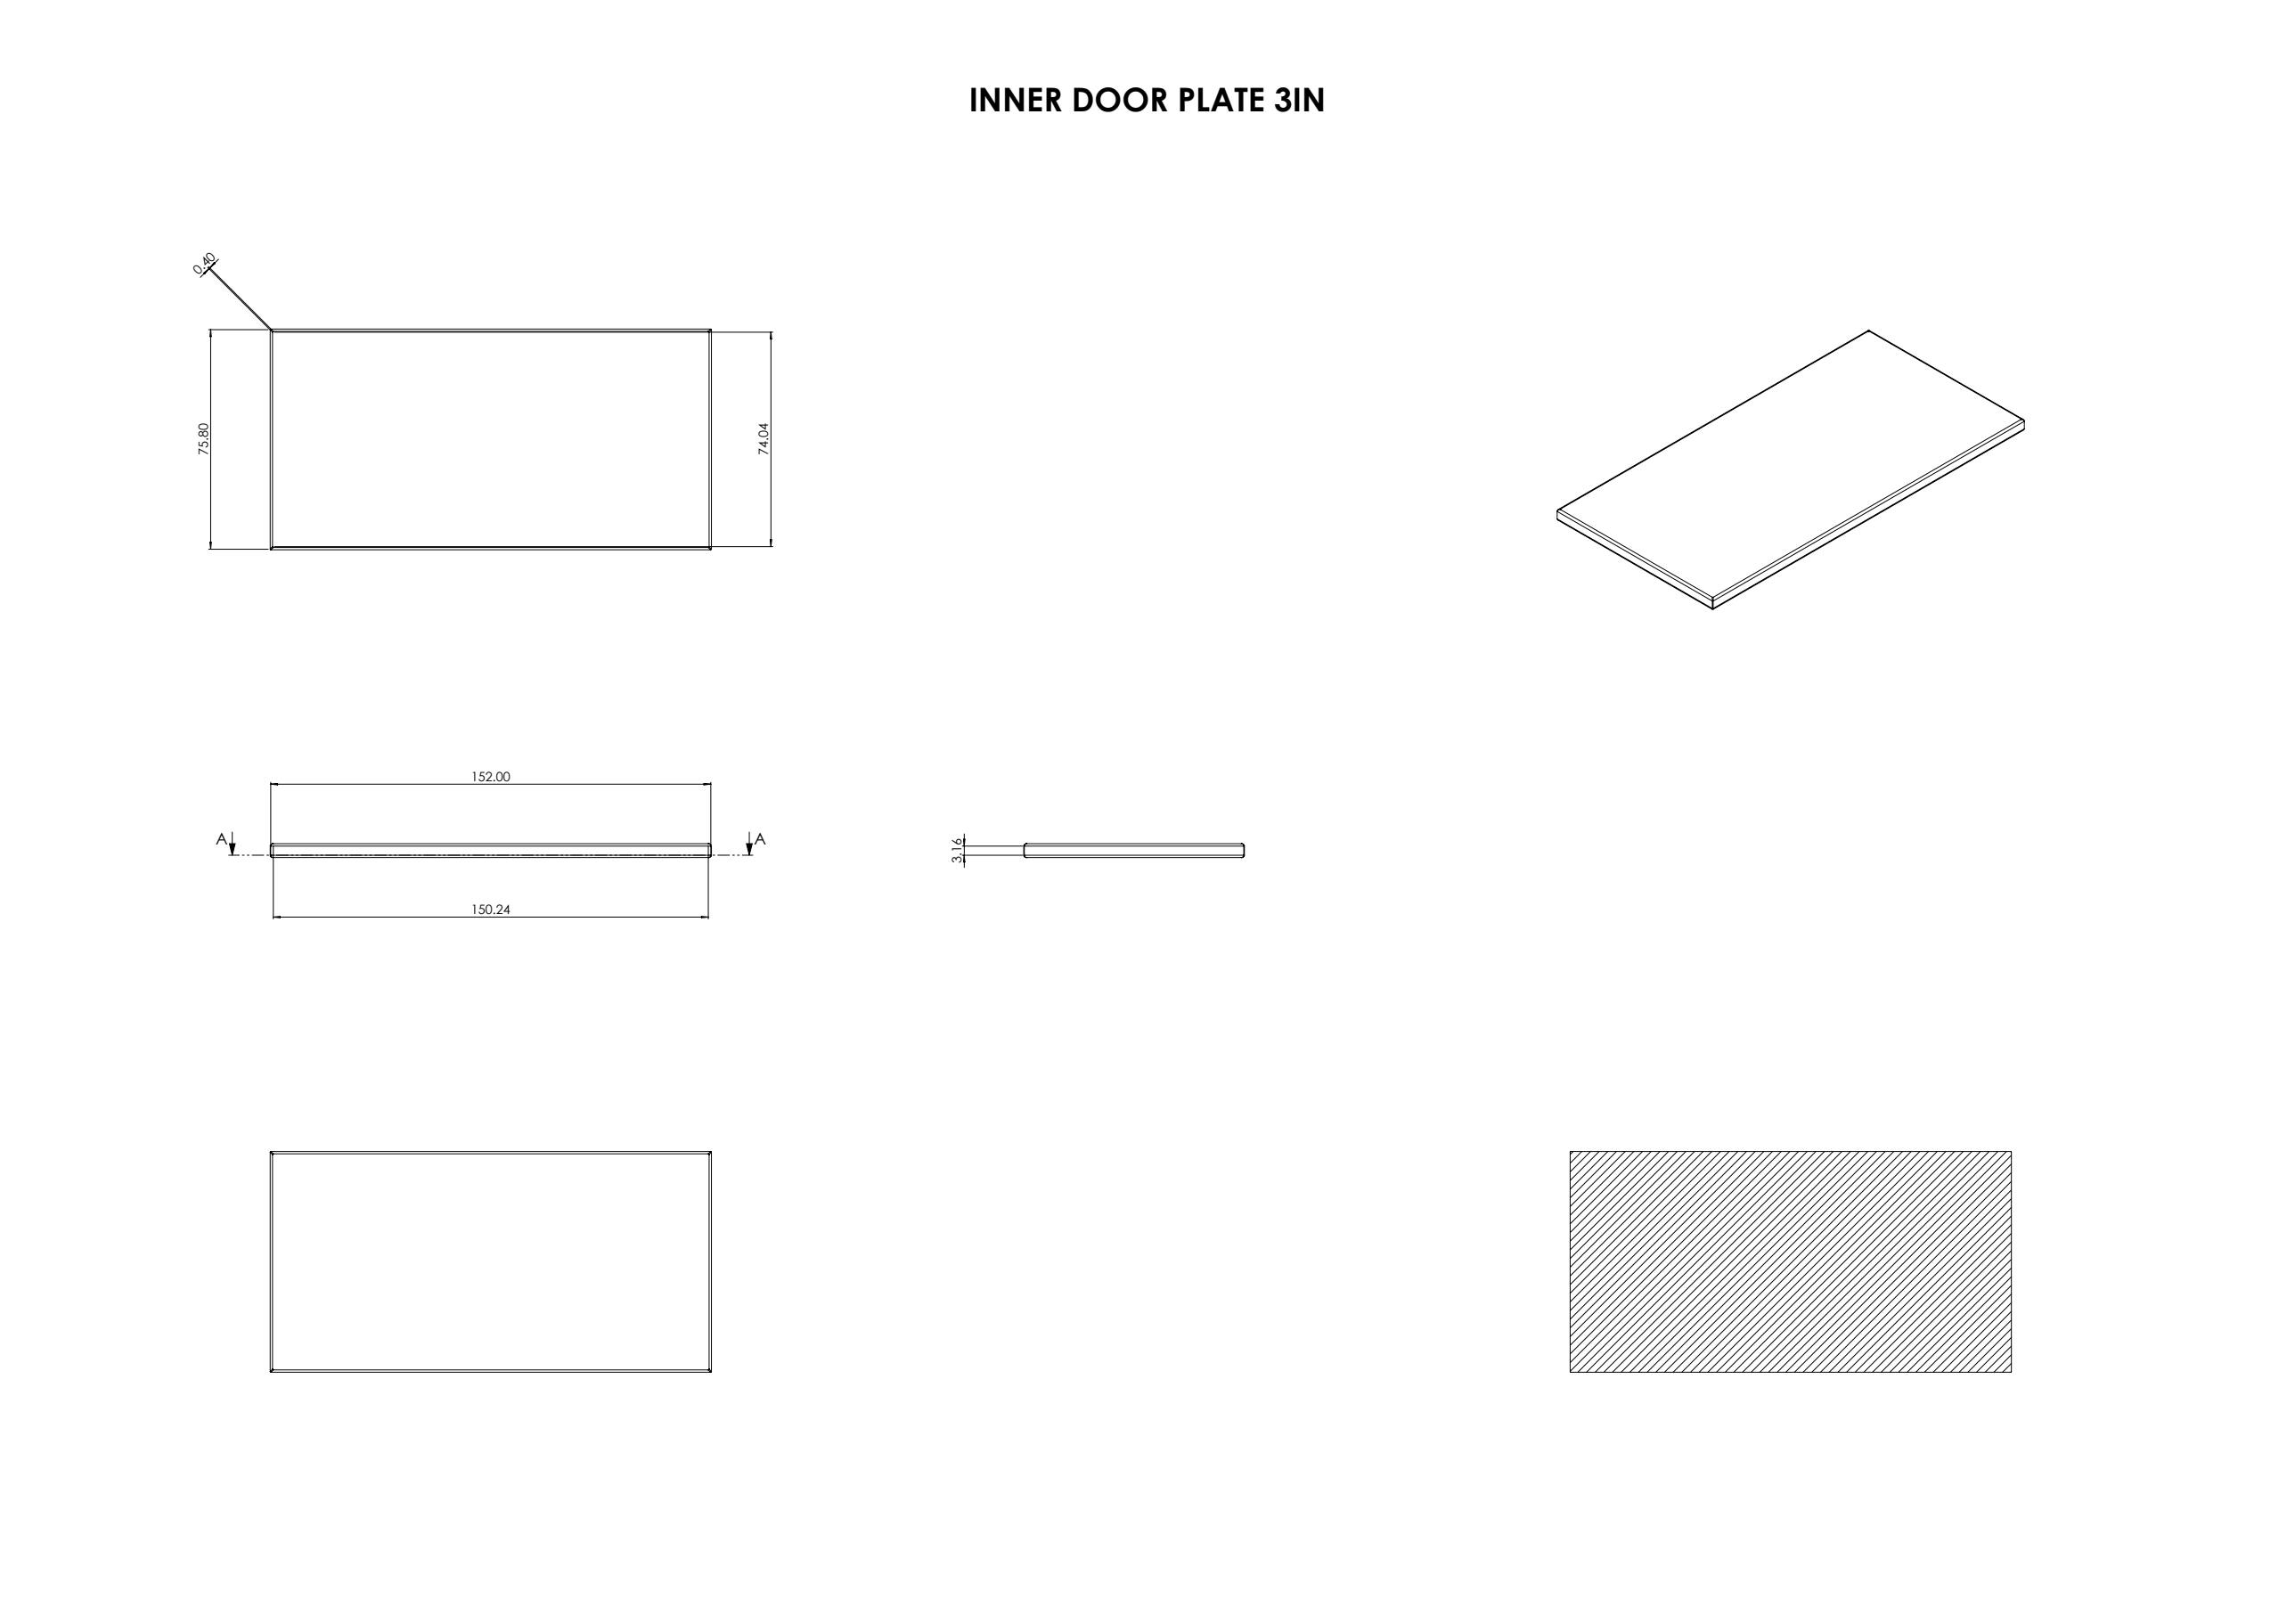
ISO-10303-21;
HEADER;
/* Generated by software containing ST-Developer
 * from STEP Tools, Inc. (www.steptools.com) 
 */

FILE_DESCRIPTION(
/* description */ (''),
/* implementation_level */ '2;1');

FILE_NAME(
/* name */ '07_Inner_Door_Plate_3in.step',
/* time_stamp */ '2026-10-25T01:30:15-07:00',
/* author */ (''),
/* organization */ (''),
/* preprocessor_version */ 'ST-DEVELOPER v20.2',
/* originating_system */ 'Autodesk Translation Framework v15.15.0.0',
/* authorisation */ '');

FILE_SCHEMA (('AUTOMOTIVE_DESIGN { 1 0 10303 214 3 1 1 }'));
ENDSEC;

DATA;
#10=MECHANICAL_DESIGN_GEOMETRIC_PRESENTATION_REPRESENTATION('',(#569),#32309);
#256=B_SPLINE_CURVE_WITH_KNOTS('',3,(#24603,#24604,#24605,#24606,#24607,
#24608,#24609,#24610,#24611,#24612,#24613,#24614,#24615,#24616,#24617,#24618,
#24619,#24620,#24621,#24622,#24623,#24624,#24625,#24626,#24627,#24628,#24629,
#24630,#24631,#24632,#24633,#24634,#24635,#24636,#24637,#24638,#24639,#24640,
#24641,#24642,#24643,#24644,#24645,#24646,#24647,#24648),.UNSPECIFIED.,
 .F.,.F.,(4,3,3,3,3,3,3,3,3,3,3,3,3,3,3,4),(0.,0.0572017311997757,0.120330894890292,
0.190833525219608,0.280000607593217,0.370000531644065,0.437396979145379,
0.498588004507602,0.56260087801746,0.634065239574647,0.727489847395828,
0.803842080523512,0.870326860317577,0.931777978339434,0.988871097236517,
1.),.UNSPECIFIED.);
#257=B_SPLINE_CURVE_WITH_KNOTS('',3,(#24650,#24651,#24652,#24653),
 .UNSPECIFIED.,.F.,.F.,(4,4),(-1.,0.),.UNSPECIFIED.);
#258=B_SPLINE_CURVE_WITH_KNOTS('',3,(#24655,#24656,#24657,#24658,#24659,
#24660,#24661,#24662,#24663,#24664,#24665,#24666,#24667,#24668,#24669,#24670,
#24671,#24672,#24673,#24674,#24675,#24676,#24677,#24678,#24679,#24680,#24681,
#24682,#24683,#24684,#24685,#24686,#24687,#24688,#24689,#24690,#24691,#24692,
#24693,#24694,#24695,#24696,#24697,#24698,#24699,#24700),.UNSPECIFIED.,
 .F.,.F.,(4,3,3,3,3,3,3,3,3,3,3,3,3,3,3,4),(0.,0.057203025224468,0.120333802338101,
0.190838689067532,0.280011837452007,0.370010357770506,0.437406670172117,
0.498598114794378,0.562610573319897,0.63407537003659,0.727505599643409,
0.803852814253569,0.870334971678201,0.931784146571509,0.988875797228613,
1.),.UNSPECIFIED.);
#259=B_SPLINE_CURVE_WITH_KNOTS('',3,(#24728,#24729,#24730,#24731,#24732,
#24733,#24734,#24735,#24736,#24737,#24738,#24739,#24740,#24741,#24742,#24743,
#24744,#24745,#24746,#24747,#24748,#24749,#24750,#24751,#24752,#24753,#24754,
#24755,#24756,#24757,#24758,#24759,#24760,#24761,#24762,#24763,#24764,#24765,
#24766,#24767,#24768,#24769,#24770,#24771,#24772,#24773),.UNSPECIFIED.,
 .F.,.F.,(4,3,3,3,3,3,3,3,3,3,3,3,3,3,3,4),(0.,0.0572017312000063,0.120330894890857,
0.190833525220496,0.280000607590238,0.370000531641458,0.437396979143437,
0.498588004432005,0.562600877937054,0.634065239482155,0.727489847253419,
0.803842080404544,0.870326860202434,0.931777978231419,0.98887109713731,
1.),.UNSPECIFIED.);
#260=B_SPLINE_CURVE_WITH_KNOTS('',3,(#24775,#24776,#24777,#24778),
 .UNSPECIFIED.,.F.,.F.,(4,4),(0.,1.),.UNSPECIFIED.);
#261=B_SPLINE_CURVE_WITH_KNOTS('',3,(#24780,#24781,#24782,#24783,#24784,
#24785,#24786,#24787,#24788,#24789,#24790,#24791,#24792,#24793,#24794,#24795,
#24796,#24797,#24798,#24799,#24800,#24801,#24802,#24803,#24804,#24805,#24806,
#24807,#24808,#24809,#24810,#24811,#24812,#24813,#24814,#24815,#24816,#24817,
#24818,#24819,#24820,#24821,#24822,#24823,#24824,#24825),.UNSPECIFIED.,
 .F.,.F.,(4,3,3,3,3,3,3,3,3,3,3,3,3,3,3,4),(0.,0.0572030252319667,0.120333802345375,
0.190838689076385,0.280011837453422,0.370010357771744,0.437406670174618,
0.498598114865344,0.562610573396659,0.634075370121406,0.727505599797859,
0.803852814376215,0.870334971791533,0.931784146677532,0.988875797332666,
1.),.UNSPECIFIED.);
#262=B_SPLINE_CURVE_WITH_KNOTS('',3,(#24852,#24853,#24854,#24855,#24856,
#24857),.UNSPECIFIED.,.F.,.F.,(4,1,1,4),(-1.70953476876622,-0.976877010723551,
-0.48843850536177,1.11854969730985E-14),.UNSPECIFIED.);
#263=B_SPLINE_CURVE_WITH_KNOTS('',3,(#24860,#24861,#24862,#24863,#24864,
#24865),.UNSPECIFIED.,.F.,.F.,(4,1,1,4),(-1.11854969730985E-14,0.48843850536177,
0.976877010723551,1.70953476876622),.UNSPECIFIED.);
#264=B_SPLINE_CURVE_WITH_KNOTS('',3,(#24900,#24901,#24902,#24903,#24904,
#24905,#24906),.UNSPECIFIED.,.F.,.F.,(4,1,1,1,4),(1.43205788482356,1.92049639018535,
2.40893489554713,2.77526377456847,3.1415926535898),.UNSPECIFIED.);
#265=B_SPLINE_CURVE_WITH_KNOTS('',3,(#24907,#24908,#24909,#24910,#24911,
#24912,#24913),.UNSPECIFIED.,.F.,.F.,(4,1,1,1,4),(-3.1415926535898,-2.77526377456847,
-2.40893489554713,-1.92049639018535,-1.43205788482356),.UNSPECIFIED.);
#266=B_SPLINE_CURVE_WITH_KNOTS('',3,(#24932,#24933,#24934,#24935,#24936,
#24937),.UNSPECIFIED.,.F.,.F.,(4,1,1,4),(-1.70953476876624,-0.976877010723567,
-0.488438505361783,0.),.UNSPECIFIED.);
#267=B_SPLINE_CURVE_WITH_KNOTS('',3,(#24938,#24939,#24940,#24941,#24942,
#24943,#24944,#24945,#24946,#24947,#24948,#24949,#24950,#24951,#24952,#24953,
#24954,#24955,#24956,#24957,#24958,#24959,#24960,#24961,#24962,#24963,#24964,
#24965,#24966,#24967,#24968,#24969,#24970,#24971,#24972,#24973,#24974,#24975,
#24976,#24977,#24978,#24979,#24980,#24981,#24982,#24983),.UNSPECIFIED.,
 .F.,.F.,(4,3,3,3,3,3,3,3,3,3,3,3,3,3,3,4),(0.,0.0572017311994344,0.120330894888931,
0.19083352521961,0.28000060759744,0.37000053164776,0.437396979149183,0.498588004127736,
0.562600877612139,0.634065239106159,0.727489846545216,0.803842079829981,
0.870326859689392,0.93177797774672,0.988871096661088,1.),.UNSPECIFIED.);
#268=B_SPLINE_CURVE_WITH_KNOTS('',3,(#24992,#24993,#24994,#24995,#24996,
#24997,#24998,#24999,#25000,#25001,#25002,#25003,#25004,#25005,#25006,#25007,
#25008,#25009,#25010,#25011,#25012,#25013,#25014,#25015,#25016,#25017,#25018,
#25019,#25020,#25021,#25022,#25023,#25024,#25025,#25026,#25027,#25028,#25029,
#25030,#25031,#25032,#25033,#25034,#25035,#25036,#25037),.UNSPECIFIED.,
 .F.,.F.,(4,3,3,3,3,3,3,3,3,3,3,3,3,3,3,4),(0.,0.0572030252313222,0.120333802345085,
0.190838689078026,0.280011837457414,0.370010357775237,0.437406670179801,
0.498598114642262,0.562610573159454,0.634075369847749,0.727505599310812,
0.803852813978605,0.870334971432735,0.931784146343715,0.988875797008993,
1.),.UNSPECIFIED.);
#269=B_SPLINE_CURVE_WITH_KNOTS('',3,(#25038,#25039,#25040,#25041,#25042,
#25043),.UNSPECIFIED.,.F.,.F.,(4,1,1,4),(0.,0.488438505361777,0.976877010723555,
1.70953476876622),.UNSPECIFIED.);
#270=B_SPLINE_CURVE_WITH_KNOTS('',3,(#25070,#25071,#25072,#25073,#25074,
#25075,#25076,#25077,#25078,#25079,#25080,#25081,#25082,#25083,#25084,#25085,
#25086,#25087,#25088,#25089,#25090,#25091,#25092,#25093,#25094,#25095,#25096,
#25097,#25098,#25099,#25100,#25101,#25102,#25103,#25104,#25105,#25106,#25107,
#25108,#25109,#25110,#25111,#25112,#25113,#25114,#25115),.UNSPECIFIED.,
 .F.,.F.,(4,3,3,3,3,3,3,3,3,3,3,3,3,3,3,4),(0.,0.0572017311976094,0.120330894887026,
0.190833525221234,0.280000607599086,0.3700005316492,0.437396979153787,0.498588004443689,
0.562600877950485,0.634065239495553,0.727489847237366,0.803842080393393,
0.87032686020045,0.931777978227553,0.988871097128439,1.),.UNSPECIFIED.);
#271=B_SPLINE_CURVE_WITH_KNOTS('',3,(#25116,#25117,#25118,#25119),
 .UNSPECIFIED.,.F.,.F.,(4,4),(0.,1.),.UNSPECIFIED.);
#272=B_SPLINE_CURVE_WITH_KNOTS('',3,(#25146,#25147,#25148,#25149),
 .UNSPECIFIED.,.F.,.F.,(4,4),(0.,1.),.UNSPECIFIED.);
#273=B_SPLINE_CURVE_WITH_KNOTS('',3,(#25150,#25151,#25152,#25153,#25154,
#25155,#25156,#25157,#25158,#25159,#25160,#25161,#25162,#25163,#25164,#25165,
#25166,#25167,#25168,#25169,#25170,#25171,#25172,#25173,#25174,#25175,#25176,
#25177,#25178,#25179,#25180,#25181,#25182,#25183,#25184,#25185,#25186,#25187,
#25188,#25189,#25190,#25191,#25192,#25193,#25194,#25195),.UNSPECIFIED.,
 .F.,.F.,(4,3,3,3,3,3,3,3,3,3,3,3,3,3,3,4),(0.,0.0572030252324622,0.120333802346723,
0.190838689076922,0.280011837457471,0.370010357775287,0.437406670183435,
0.498598114641987,0.562610573159151,0.634075369845933,0.727505599300381,
0.803852813971137,0.870334971421258,0.931784146332158,0.988875796999179,
1.),.UNSPECIFIED.);
#274=B_SPLINE_CURVE_WITH_KNOTS('',3,(#25222,#25223,#25224,#25225,#25226,
#25227),.UNSPECIFIED.,.F.,.F.,(4,1,1,4),(0.,0.488438505361783,0.976877010723567,
1.70953476876624),.UNSPECIFIED.);
#275=B_SPLINE_CURVE_WITH_KNOTS('',3,(#25256,#25257,#25258,#25259,#25260,
#25261),.UNSPECIFIED.,.F.,.F.,(4,1,1,4),(-1.70953476876622,-0.976877010723555,
-0.488438505361777,0.),.UNSPECIFIED.);
#276=B_SPLINE_CURVE_WITH_KNOTS('',3,(#25287,#25288,#25289,#25290,#25291,
#25292,#25293,#25294,#25295,#25296,#25297,#25298,#25299,#25300,#25301,#25302,
#25303,#25304,#25305,#25306,#25307,#25308,#25309,#25310,#25311,#25312,#25313,
#25314,#25315,#25316,#25317,#25318,#25319,#25320,#25321,#25322,#25323,#25324,
#25325,#25326,#25327,#25328,#25329,#25330,#25331,#25332),.UNSPECIFIED.,
 .F.,.F.,(4,3,3,3,3,3,3,3,3,3,3,3,3,3,3,4),(0.,0.0572017311991183,0.120330894889653,
0.190833525219955,0.280000607594411,0.37000053164511,0.437396979144203,
0.498588004649256,0.56260087816826,0.634065239749291,0.727489847706123,
0.803842080776209,0.870326860547973,0.931777978552727,0.988871097444316,
1.),.UNSPECIFIED.);
#277=B_SPLINE_CURVE_WITH_KNOTS('',3,(#25334,#25335,#25336,#25337),
 .UNSPECIFIED.,.F.,.F.,(4,4),(0.,1.),.UNSPECIFIED.);
#278=B_SPLINE_CURVE_WITH_KNOTS('',3,(#25338,#25339,#25340,#25341,#25342,
#25343,#25344,#25345,#25346,#25347,#25348,#25349,#25350,#25351,#25352,#25353,
#25354,#25355,#25356,#25357,#25358,#25359,#25360,#25361,#25362,#25363,#25364,
#25365,#25366,#25367,#25368,#25369,#25370,#25371,#25372,#25373,#25374,#25375,
#25376,#25377,#25378,#25379,#25380,#25381,#25382,#25383),.UNSPECIFIED.,
 .F.,.F.,(4,3,3,3,3,3,3,3,3,3,3,3,3,3,3,4),(0.,0.0572030252343024,0.12033380234866,
0.190838689076873,0.280011837448138,0.370010357767121,0.437406670172275,
0.498598114697011,0.562610573216881,0.634075369917583,0.727505599449089,
0.803852814091775,0.870334971532607,0.931784146442687,0.988875797099411,
1.),.UNSPECIFIED.);
#279=B_SPLINE_CURVE_WITH_KNOTS('',3,(#25410,#25411,#25412,#25413,#25414,
#25415,#25416,#25417,#25418,#25419,#25420,#25421,#25422,#25423,#25424,#25425,
#25426,#25427,#25428,#25429,#25430,#25431,#25432,#25433,#25434,#25435,#25436,
#25437,#25438,#25439,#25440,#25441,#25442,#25443,#25444,#25445,#25446,#25447,
#25448,#25449,#25450,#25451,#25452,#25453,#25454,#25455),.UNSPECIFIED.,
 .F.,.F.,(4,3,3,3,3,3,3,3,3,3,3,3,3,3,3,4),(0.,0.0572017312009936,0.120330894888744,
0.190833525225305,0.280000607597786,0.370000531648063,0.437396979151322,
0.49858800483577,0.562600878367579,0.634065239978569,0.727489848107998,
0.8038420811056,0.870326860843456,0.931777978817204,0.988871097702708,1.),
 .UNSPECIFIED.);
#280=B_SPLINE_CURVE_WITH_KNOTS('',3,(#25457,#25458,#25459,#25460),
 .UNSPECIFIED.,.F.,.F.,(4,4),(0.,1.),.UNSPECIFIED.);
#281=B_SPLINE_CURVE_WITH_KNOTS('',3,(#25462,#25463,#25464,#25465,#25466,
#25467,#25468,#25469,#25470,#25471,#25472,#25473,#25474,#25475,#25476,#25477,
#25478,#25479,#25480,#25481,#25482,#25483,#25484,#25485,#25486,#25487,#25488,
#25489,#25490,#25491,#25492,#25493,#25494,#25495,#25496,#25497,#25498,#25499,
#25500,#25501,#25502,#25503,#25504,#25505,#25506,#25507),.UNSPECIFIED.,
 .F.,.F.,(4,3,3,3,3,3,3,3,3,3,3,3,3,3,3,4),(0.,0.0572030252317164,0.120333802345145,
0.19083868907559,0.280011837455817,0.37001035777384,0.437406670175968,0.498598114641638,
0.562610573158253,0.634075369846188,0.727505599314327,0.803852813981206,
0.870334971433397,0.93178414634131,0.98887579700713,1.),.UNSPECIFIED.);
#282=B_SPLINE_CURVE_WITH_KNOTS('',3,(#25534,#25535,#25536,#25537,#25538,
#25539),.UNSPECIFIED.,.F.,.F.,(4,1,1,4),(-1.70953476876621,-0.976877010723542,
-0.48843850536176,2.22044604925035E-14),.UNSPECIFIED.);
#283=B_SPLINE_CURVE_WITH_KNOTS('',3,(#25542,#25543,#25544,#25545,#25546,
#25547),.UNSPECIFIED.,.F.,.F.,(4,1,1,4),(-2.22044604925035E-14,0.48843850536176,
0.976877010723542,1.70953476876621),.UNSPECIFIED.);
#284=B_SPLINE_CURVE_WITH_KNOTS('',3,(#25578,#25579,#25580,#25581,#25582,
#25583),.UNSPECIFIED.,.F.,.F.,(4,1,1,4),(-1.70953476876621,-0.97687701072354,
-0.488438505361759,2.22044604925031E-14),.UNSPECIFIED.);
#285=B_SPLINE_CURVE_WITH_KNOTS('',3,(#25584,#25585,#25586,#25587,#25588,
#25589),.UNSPECIFIED.,.F.,.F.,(4,1,1,4),(-2.22044604925031E-14,0.488438505361759,
0.97687701072354,1.70953476876621),.UNSPECIFIED.);
#286=B_SPLINE_CURVE_WITH_KNOTS('',3,(#25594,#25595,#25596,#25597,#25598,
#25599),.UNSPECIFIED.,.F.,.F.,(4,1,1,4),(-1.70953476876623,-0.976877010723559,
-0.488438505361781,-2.77555756156289E-15),.UNSPECIFIED.);
#287=B_SPLINE_CURVE_WITH_KNOTS('',3,(#25600,#25601,#25602,#25603,#25604,
#25605,#25606,#25607,#25608,#25609,#25610,#25611,#25612,#25613,#25614,#25615,
#25616,#25617,#25618,#25619,#25620,#25621,#25622,#25623,#25624,#25625,#25626,
#25627,#25628,#25629,#25630,#25631,#25632,#25633,#25634,#25635,#25636,#25637,
#25638,#25639,#25640,#25641,#25642,#25643,#25644,#25645),.UNSPECIFIED.,
 .F.,.F.,(4,3,3,3,3,3,3,3,3,3,3,3,3,3,3,4),(0.,0.0572017311987612,0.120330894889715,
0.190833525218877,0.280000607593098,0.370000531643961,0.437396979144952,
0.498588004371557,0.562600877871927,0.634065239405833,0.727489847083102,
0.803842080268102,0.870326860085879,0.931777978122396,0.988871097026644,
1.),.UNSPECIFIED.);
#288=B_SPLINE_CURVE_WITH_KNOTS('',3,(#25654,#25655,#25656,#25657,#25658,
#25659,#25660,#25661,#25662,#25663,#25664,#25665,#25666,#25667,#25668,#25669,
#25670,#25671,#25672,#25673,#25674,#25675,#25676,#25677,#25678,#25679,#25680,
#25681,#25682,#25683,#25684,#25685,#25686,#25687,#25688,#25689,#25690,#25691,
#25692,#25693,#25694,#25695,#25696,#25697,#25698,#25699),.UNSPECIFIED.,
 .F.,.F.,(4,3,3,3,3,3,3,3,3,3,3,3,3,3,3,4),(0.,0.0572030252318266,0.120333802345496,
0.190838689075676,0.280011837456741,0.370010357774648,0.437406670177162,
0.498598114850172,0.562610573381775,0.634075370104953,0.727505599770209,
0.803852814352912,0.870334971770891,0.9317841466576,0.988875797314384,1.),
 .UNSPECIFIED.);
#289=B_SPLINE_CURVE_WITH_KNOTS('',3,(#25700,#25701,#25702,#25703,#25704,
#25705),.UNSPECIFIED.,.F.,.F.,(4,1,1,4),(2.77555756156289E-15,0.488438505361782,
0.976877010723562,1.70953476876623),.UNSPECIFIED.);
#290=B_SPLINE_CURVE_WITH_KNOTS('',3,(#25736,#25737,#25738,#25739),
 .UNSPECIFIED.,.F.,.F.,(4,4),(0.,1.),.UNSPECIFIED.);
#291=B_SPLINE_CURVE_WITH_KNOTS('',3,(#25740,#25741,#25742,#25743,#25744,
#25745,#25746,#25747,#25748,#25749,#25750,#25751,#25752,#25753,#25754,#25755,
#25756,#25757,#25758,#25759,#25760,#25761,#25762,#25763,#25764,#25765,#25766,
#25767,#25768,#25769,#25770,#25771,#25772,#25773,#25774,#25775,#25776,#25777,
#25778,#25779,#25780,#25781,#25782,#25783,#25784,#25785),.UNSPECIFIED.,
 .F.,.F.,(4,3,3,3,3,3,3,3,3,3,3,3,3,3,3,4),(0.,0.0572030252318119,0.120333802345044,
0.190838689074226,0.280011837457671,0.370010357775463,0.437406670175368,
0.498598114719374,0.562610573241369,0.634075369941395,0.727505599476499,
0.803852814114293,0.870334971552934,0.931784146453147,0.98887579711519,
1.),.UNSPECIFIED.);
#292=B_SPLINE_CURVE_WITH_KNOTS('',3,(#25811,#25812,#25813,#25814,#25815,
#25816,#25817,#25818,#25819,#25820,#25821,#25822,#25823,#25824,#25825,#25826,
#25827,#25828,#25829,#25830,#25831,#25832,#25833,#25834,#25835,#25836,#25837,
#25838,#25839,#25840,#25841,#25842,#25843,#25844,#25845,#25846,#25847,#25848,
#25849,#25850,#25851,#25852,#25853,#25854,#25855,#25856),.UNSPECIFIED.,
 .F.,.F.,(4,3,3,3,3,3,3,3,3,3,3,3,3,3,3,4),(0.,0.0572017311987599,0.120330894889451,
0.190833525224185,0.28000060760209,0.370000531651829,0.437396979150436,
0.498588004343821,0.562600877842339,0.63406523937154,0.727489847024129,
0.803842080219329,0.870326860044885,0.931777978082536,0.988871096986048,
1.),.UNSPECIFIED.);
#293=B_SPLINE_CURVE_WITH_KNOTS('',3,(#25857,#25858,#25859,#25860),
 .UNSPECIFIED.,.F.,.F.,(4,4),(0.,1.),.UNSPECIFIED.);
#294=B_SPLINE_CURVE_WITH_KNOTS('',3,(#25886,#25887,#25888,#25889,#25890,
#25891),.UNSPECIFIED.,.F.,.F.,(4,1,1,4),(-1.70953476876623,-0.976877010723562,
-0.488438505361782,-2.77555756156289E-15),.UNSPECIFIED.);
#295=B_SPLINE_CURVE_WITH_KNOTS('',3,(#25921,#25922,#25923,#25924,#25925,
#25926),.UNSPECIFIED.,.F.,.F.,(4,1,1,4),(2.77555756156289E-15,0.488438505361781,
0.976877010723559,1.70953476876623),.UNSPECIFIED.);
#471=B_SPLINE_SURFACE_WITH_KNOTS('',3,3,((#24577,#24578,#24579,#24580,#24581,
#24582),(#24583,#24584,#24585,#24586,#24587,#24588),(#24589,#24590,#24591,
#24592,#24593,#24594),(#24595,#24596,#24597,#24598,#24599,#24600)),
 .UNSPECIFIED.,.F.,.F.,.F.,(4,4),(4,1,1,4),(0.,1.),(0.,0.571428571428571,
0.857142857142857,1.),.UNSPECIFIED.);
#472=B_SPLINE_SURFACE_WITH_KNOTS('',3,3,((#24702,#24703,#24704,#24705,#24706,
#24707),(#24708,#24709,#24710,#24711,#24712,#24713),(#24714,#24715,#24716,
#24717,#24718,#24719),(#24720,#24721,#24722,#24723,#24724,#24725)),
 .UNSPECIFIED.,.F.,.F.,.F.,(4,4),(4,1,1,4),(0.,1.),(0.,0.571428571428571,
0.857142857142857,1.),.UNSPECIFIED.);
#473=B_SPLINE_SURFACE_WITH_KNOTS('',3,3,((#24827,#24828,#24829,#24830,#24831,
#24832),(#24833,#24834,#24835,#24836,#24837,#24838),(#24839,#24840,#24841,
#24842,#24843,#24844),(#24845,#24846,#24847,#24848,#24849,#24850)),
 .UNSPECIFIED.,.F.,.F.,.F.,(4,4),(4,1,1,4),(0.,1.),(-1.70953476876622,-0.976877010723551,
-0.48843850536177,1.11854969730985E-14),.UNSPECIFIED.);
#474=B_SPLINE_SURFACE_WITH_KNOTS('',3,3,((#24872,#24873,#24874,#24875,#24876,
#24877,#24878),(#24879,#24880,#24881,#24882,#24883,#24884,#24885),(#24886,
#24887,#24888,#24889,#24890,#24891,#24892),(#24893,#24894,#24895,#24896,
#24897,#24898,#24899)),.UNSPECIFIED.,.F.,.F.,.F.,(4,4),(4,1,1,1,4),(0.,
1.),(-3.1415926535898,-2.77526377456847,-2.40893489554713,-1.92049639018535,
-1.43205788482356),.UNSPECIFIED.);
#475=B_SPLINE_SURFACE_WITH_KNOTS('',3,3,((#25044,#25045,#25046,#25047,#25048,
#25049),(#25050,#25051,#25052,#25053,#25054,#25055),(#25056,#25057,#25058,
#25059,#25060,#25061),(#25062,#25063,#25064,#25065,#25066,#25067)),
 .UNSPECIFIED.,.F.,.F.,.F.,(4,4),(4,1,1,4),(0.,1.),(0.,0.571428571428571,
0.857142857142857,1.),.UNSPECIFIED.);
#476=B_SPLINE_SURFACE_WITH_KNOTS('',3,3,((#25121,#25122,#25123,#25124,#25125,
#25126),(#25127,#25128,#25129,#25130,#25131,#25132),(#25133,#25134,#25135,
#25136,#25137,#25138),(#25139,#25140,#25141,#25142,#25143,#25144)),
 .UNSPECIFIED.,.F.,.F.,.F.,(4,4),(4,1,1,4),(0.,1.),(0.,0.571428571428571,
0.857142857142857,1.),.UNSPECIFIED.);
#477=B_SPLINE_SURFACE_WITH_KNOTS('',3,3,((#25196,#25197,#25198,#25199,#25200,
#25201),(#25202,#25203,#25204,#25205,#25206,#25207),(#25208,#25209,#25210,
#25211,#25212,#25213),(#25214,#25215,#25216,#25217,#25218,#25219)),
 .UNSPECIFIED.,.F.,.F.,.F.,(4,4),(4,1,1,4),(0.,1.),(-1.70953476876624,-0.976877010723567,
-0.488438505361783,0.),.UNSPECIFIED.);
#478=B_SPLINE_SURFACE_WITH_KNOTS('',3,3,((#25232,#25233,#25234,#25235,#25236,
#25237),(#25238,#25239,#25240,#25241,#25242,#25243),(#25244,#25245,#25246,
#25247,#25248,#25249),(#25250,#25251,#25252,#25253,#25254,#25255)),
 .UNSPECIFIED.,.F.,.F.,.F.,(4,4),(4,1,1,4),(0.,1.),(-1.70953476876622,-0.976877010723555,
-0.488438505361777,0.),.UNSPECIFIED.);
#479=B_SPLINE_SURFACE_WITH_KNOTS('',3,3,((#25262,#25263,#25264,#25265,#25266,
#25267),(#25268,#25269,#25270,#25271,#25272,#25273),(#25274,#25275,#25276,
#25277,#25278,#25279),(#25280,#25281,#25282,#25283,#25284,#25285)),
 .UNSPECIFIED.,.F.,.F.,.F.,(4,4),(4,1,1,4),(0.,1.),(0.,0.571428571428571,
0.857142857142857,1.),.UNSPECIFIED.);
#480=B_SPLINE_SURFACE_WITH_KNOTS('',3,3,((#25384,#25385,#25386,#25387,#25388,
#25389),(#25390,#25391,#25392,#25393,#25394,#25395),(#25396,#25397,#25398,
#25399,#25400,#25401),(#25402,#25403,#25404,#25405,#25406,#25407)),
 .UNSPECIFIED.,.F.,.F.,.F.,(4,4),(4,1,1,4),(0.,1.),(0.,0.571428571428571,
0.857142857142857,1.),.UNSPECIFIED.);
#481=B_SPLINE_SURFACE_WITH_KNOTS('',3,3,((#25509,#25510,#25511,#25512,#25513,
#25514),(#25515,#25516,#25517,#25518,#25519,#25520),(#25521,#25522,#25523,
#25524,#25525,#25526),(#25527,#25528,#25529,#25530,#25531,#25532)),
 .UNSPECIFIED.,.F.,.F.,.F.,(4,4),(4,1,1,4),(0.,1.),(-1.70953476876621,-0.976877010723542,
-0.48843850536176,2.22044604925035E-14),.UNSPECIFIED.);
#482=B_SPLINE_SURFACE_WITH_KNOTS('',3,3,((#25554,#25555,#25556,#25557,#25558,
#25559),(#25560,#25561,#25562,#25563,#25564,#25565),(#25566,#25567,#25568,
#25569,#25570,#25571),(#25572,#25573,#25574,#25575,#25576,#25577)),
 .UNSPECIFIED.,.F.,.F.,.F.,(4,4),(4,1,1,4),(0.,1.),(-1.70953476876621,-0.97687701072354,
-0.488438505361759,2.22044604925031E-14),.UNSPECIFIED.);
#483=B_SPLINE_SURFACE_WITH_KNOTS('',3,3,((#25711,#25712,#25713,#25714,#25715,
#25716),(#25717,#25718,#25719,#25720,#25721,#25722),(#25723,#25724,#25725,
#25726,#25727,#25728),(#25729,#25730,#25731,#25732,#25733,#25734)),
 .UNSPECIFIED.,.F.,.F.,.F.,(4,4),(4,1,1,4),(0.,1.),(0.,0.571428571428571,
0.857142857142857,1.),.UNSPECIFIED.);
#484=B_SPLINE_SURFACE_WITH_KNOTS('',3,3,((#25786,#25787,#25788,#25789,#25790,
#25791),(#25792,#25793,#25794,#25795,#25796,#25797),(#25798,#25799,#25800,
#25801,#25802,#25803),(#25804,#25805,#25806,#25807,#25808,#25809)),
 .UNSPECIFIED.,.F.,.F.,.F.,(4,4),(4,1,1,4),(0.,1.),(0.,0.571428571428571,
0.857142857142857,1.),.UNSPECIFIED.);
#485=B_SPLINE_SURFACE_WITH_KNOTS('',3,3,((#25861,#25862,#25863,#25864,#25865,
#25866),(#25867,#25868,#25869,#25870,#25871,#25872),(#25873,#25874,#25875,
#25876,#25877,#25878),(#25879,#25880,#25881,#25882,#25883,#25884)),
 .UNSPECIFIED.,.F.,.F.,.F.,(4,4),(4,1,1,4),(0.,1.),(-1.70953476876623,-0.976877010723562,
-0.488438505361782,-2.77555756156289E-15),.UNSPECIFIED.);
#486=B_SPLINE_SURFACE_WITH_KNOTS('',3,3,((#25897,#25898,#25899,#25900,#25901,
#25902),(#25903,#25904,#25905,#25906,#25907,#25908),(#25909,#25910,#25911,
#25912,#25913,#25914),(#25915,#25916,#25917,#25918,#25919,#25920)),
 .UNSPECIFIED.,.F.,.F.,.F.,(4,4),(4,1,1,4),(0.,1.),(-1.70953476876623,-0.976877010723559,
-0.488438505361781,-2.77555756156289E-15),.UNSPECIFIED.);
#541=SHAPE_REPRESENTATION_RELATIONSHIP('SRR','None',#32368,#555);
#555=ADVANCED_BREP_SHAPE_REPRESENTATION('',(#583),#32301);
#569=STYLED_ITEM('',(#32495),#583);
#583=MANIFOLD_SOLID_BREP('Body1',#13810);
#718=CYLINDRICAL_SURFACE('',#14416,0.8);
#719=CYLINDRICAL_SURFACE('',#14418,0.8);
#720=CYLINDRICAL_SURFACE('',#14421,0.8);
#721=CYLINDRICAL_SURFACE('',#14423,0.8);
#722=CYLINDRICAL_SURFACE('',#14426,0.8);
#723=CYLINDRICAL_SURFACE('',#14428,0.8);
#724=CYLINDRICAL_SURFACE('',#14429,0.8);
#725=CYLINDRICAL_SURFACE('',#14431,0.8);
#1561=FACE_OUTER_BOUND('',#2396,.T.);
#1562=FACE_OUTER_BOUND('',#2397,.T.);
#1563=FACE_OUTER_BOUND('',#2398,.T.);
#1564=FACE_OUTER_BOUND('',#2399,.T.);
#1565=FACE_OUTER_BOUND('',#2400,.T.);
#1566=FACE_OUTER_BOUND('',#2401,.T.);
#1567=FACE_OUTER_BOUND('',#2402,.T.);
#1568=FACE_OUTER_BOUND('',#2403,.T.);
#1569=FACE_OUTER_BOUND('',#2404,.T.);
#1570=FACE_OUTER_BOUND('',#2405,.T.);
#1571=FACE_OUTER_BOUND('',#2406,.T.);
#1572=FACE_OUTER_BOUND('',#2407,.T.);
#1573=FACE_OUTER_BOUND('',#2408,.T.);
#1574=FACE_OUTER_BOUND('',#2409,.T.);
#1575=FACE_OUTER_BOUND('',#2410,.T.);
#1576=FACE_OUTER_BOUND('',#2411,.T.);
#1577=FACE_OUTER_BOUND('',#2412,.T.);
#1578=FACE_OUTER_BOUND('',#2413,.T.);
#1579=FACE_OUTER_BOUND('',#2414,.T.);
#1580=FACE_OUTER_BOUND('',#2415,.T.);
#1581=FACE_OUTER_BOUND('',#2416,.T.);
#1582=FACE_OUTER_BOUND('',#2417,.T.);
#1583=FACE_OUTER_BOUND('',#2418,.T.);
#1584=FACE_OUTER_BOUND('',#2419,.T.);
#1585=FACE_OUTER_BOUND('',#2420,.T.);
#1586=FACE_OUTER_BOUND('',#2421,.T.);
#1587=FACE_OUTER_BOUND('',#2422,.T.);
#1588=FACE_OUTER_BOUND('',#2423,.T.);
#1589=FACE_OUTER_BOUND('',#2424,.T.);
#1590=FACE_OUTER_BOUND('',#2425,.T.);
#1591=FACE_OUTER_BOUND('',#2426,.T.);
#1592=FACE_OUTER_BOUND('',#2427,.T.);
#1593=FACE_OUTER_BOUND('',#2428,.T.);
#1594=FACE_OUTER_BOUND('',#2429,.T.);
#2396=EDGE_LOOP('',(#10209,#10210,#10211,#10212));
#2397=EDGE_LOOP('',(#10213,#10214,#10215,#10216));
#2398=EDGE_LOOP('',(#10217,#10218,#10219,#10220));
#2399=EDGE_LOOP('',(#10221,#10222,#10223,#10224));
#2400=EDGE_LOOP('',(#10225,#10226,#10227,#10228));
#2401=EDGE_LOOP('',(#10229,#10230,#10231,#10232,#10233,#10234,#10235,#10236));
#2402=EDGE_LOOP('',(#10237,#10238,#10239,#10240,#10241,#10242));
#2403=EDGE_LOOP('',(#10243,#10244,#10245,#10246));
#2404=EDGE_LOOP('',(#10247,#10248,#10249,#10250,#10251,#10252));
#2405=EDGE_LOOP('',(#10253,#10254,#10255,#10256));
#2406=EDGE_LOOP('',(#10257,#10258,#10259,#10260));
#2407=EDGE_LOOP('',(#10261,#10262,#10263,#10264));
#2408=EDGE_LOOP('',(#10265,#10266,#10267,#10268));
#2409=EDGE_LOOP('',(#10269,#10270,#10271,#10272));
#2410=EDGE_LOOP('',(#10273,#10274,#10275,#10276));
#2411=EDGE_LOOP('',(#10277,#10278,#10279,#10280));
#2412=EDGE_LOOP('',(#10281,#10282,#10283,#10284));
#2413=EDGE_LOOP('',(#10285,#10286,#10287,#10288));
#2414=EDGE_LOOP('',(#10289,#10290,#10291,#10292));
#2415=EDGE_LOOP('',(#10293,#10294,#10295,#10296,#10297,#10298));
#2416=EDGE_LOOP('',(#10299,#10300,#10301,#10302));
#2417=EDGE_LOOP('',(#10303,#10304,#10305,#10306,#10307,#10308));
#2418=EDGE_LOOP('',(#10309,#10310,#10311,#10312,#10313,#10314,#10315,#10316));
#2419=EDGE_LOOP('',(#10317,#10318,#10319,#10320));
#2420=EDGE_LOOP('',(#10321,#10322,#10323,#10324));
#2421=EDGE_LOOP('',(#10325,#10326,#10327,#10328));
#2422=EDGE_LOOP('',(#10329,#10330,#10331,#10332));
#2423=EDGE_LOOP('',(#10333,#10334,#10335,#10336));
#2424=EDGE_LOOP('',(#10337,#10338,#10339,#10340,#10341,#10342));
#2425=EDGE_LOOP('',(#10343,#10344,#10345,#10346));
#2426=EDGE_LOOP('',(#10347,#10348,#10349,#10350,#10351,#10352));
#2427=EDGE_LOOP('',(#10353,#10354,#10355,#10356,#10357,#10358));
#2428=EDGE_LOOP('',(#10359,#10360,#10361,#10362));
#2429=EDGE_LOOP('',(#10363,#10364,#10365,#10366,#10367,#10368));
#3315=LINE('',#24701,#4626);
#3316=LINE('',#24826,#4627);
#3317=LINE('',#24859,#4628);
#3318=LINE('',#24868,#4629);
#3319=LINE('',#24870,#4630);
#3320=LINE('',#24871,#4631);
#3321=LINE('',#24916,#4632);
#3322=LINE('',#24918,#4633);
#3323=LINE('',#24920,#4634);
#3324=LINE('',#24922,#4635);
#3325=LINE('',#24924,#4636);
#3326=LINE('',#24926,#4637);
#3327=LINE('',#24927,#4638);
#3328=LINE('',#24930,#4639);
#3329=LINE('',#24986,#4640);
#3330=LINE('',#24987,#4641);
#3331=LINE('',#24990,#4642);
#3332=LINE('',#25120,#4643);
#3333=LINE('',#25221,#4644);
#3334=LINE('',#25230,#4645);
#3335=LINE('',#25231,#4646);
#3336=LINE('',#25508,#4647);
#3337=LINE('',#25541,#4648);
#3338=LINE('',#25550,#4649);
#3339=LINE('',#25552,#4650);
#3340=LINE('',#25553,#4651);
#3341=LINE('',#25592,#4652);
#3342=LINE('',#25648,#4653);
#3343=LINE('',#25649,#4654);
#3344=LINE('',#25652,#4655);
#3345=LINE('',#25708,#4656);
#3346=LINE('',#25709,#4657);
#3347=LINE('',#25710,#4658);
#3348=LINE('',#25892,#4659);
#3349=LINE('',#25895,#4660);
#3350=LINE('',#25896,#4661);
#3351=LINE('',#25928,#4662);
#3352=LINE('',#25930,#4663);
#3353=LINE('',#25933,#4664);
#3354=LINE('',#25935,#4665);
#4626=VECTOR('',#16305,10.);
#4627=VECTOR('',#16306,10.);
#4628=VECTOR('',#16307,10.);
#4629=VECTOR('',#16310,10.);
#4630=VECTOR('',#16311,10.);
#4631=VECTOR('',#16312,10.);
#4632=VECTOR('',#16315,10.);
#4633=VECTOR('',#16316,10.);
#4634=VECTOR('',#16317,10.);
#4635=VECTOR('',#16318,10.);
#4636=VECTOR('',#16319,10.);
#4637=VECTOR('',#16320,10.);
#4638=VECTOR('',#16321,10.);
#4639=VECTOR('',#16324,10.);
#4640=VECTOR('',#16327,10.);
#4641=VECTOR('',#16328,10.);
#4642=VECTOR('',#16331,10.);
#4643=VECTOR('',#16332,10.);
#4644=VECTOR('',#16333,10.);
#4645=VECTOR('',#16336,10.);
#4646=VECTOR('',#16337,10.);
#4647=VECTOR('',#16338,10.);
#4648=VECTOR('',#16339,10.);
#4649=VECTOR('',#16342,10.);
#4650=VECTOR('',#16343,10.);
#4651=VECTOR('',#16344,10.);
#4652=VECTOR('',#16347,10.);
#4653=VECTOR('',#16350,10.);
#4654=VECTOR('',#16351,10.);
#4655=VECTOR('',#16354,10.);
#4656=VECTOR('',#16357,10.);
#4657=VECTOR('',#16358,10.);
#4658=VECTOR('',#16359,10.);
#4659=VECTOR('',#16360,10.);
#4660=VECTOR('',#16363,10.);
#4661=VECTOR('',#16364,10.);
#4662=VECTOR('',#16367,10.);
#4663=VECTOR('',#16370,10.);
#4664=VECTOR('',#16375,10.);
#4665=VECTOR('',#16378,10.);
#5976=VERTEX_POINT('',#24601);
#5977=VERTEX_POINT('',#24602);
#5978=VERTEX_POINT('',#24649);
#5979=VERTEX_POINT('',#24654);
#5980=VERTEX_POINT('',#24726);
#5981=VERTEX_POINT('',#24727);
#5982=VERTEX_POINT('',#24774);
#5983=VERTEX_POINT('',#24779);
#5984=VERTEX_POINT('',#24851);
#5985=VERTEX_POINT('',#24858);
#5986=VERTEX_POINT('',#24867);
#5987=VERTEX_POINT('',#24869);
#5988=VERTEX_POINT('',#24915);
#5989=VERTEX_POINT('',#24917);
#5990=VERTEX_POINT('',#24919);
#5991=VERTEX_POINT('',#24921);
#5992=VERTEX_POINT('',#24923);
#5993=VERTEX_POINT('',#24925);
#5994=VERTEX_POINT('',#24929);
#5995=VERTEX_POINT('',#24931);
#5996=VERTEX_POINT('',#24985);
#5997=VERTEX_POINT('',#24989);
#5998=VERTEX_POINT('',#24991);
#5999=VERTEX_POINT('',#25068);
#6000=VERTEX_POINT('',#25069);
#6001=VERTEX_POINT('',#25145);
#6002=VERTEX_POINT('',#25220);
#6003=VERTEX_POINT('',#25229);
#6004=VERTEX_POINT('',#25286);
#6005=VERTEX_POINT('',#25333);
#6006=VERTEX_POINT('',#25408);
#6007=VERTEX_POINT('',#25409);
#6008=VERTEX_POINT('',#25456);
#6009=VERTEX_POINT('',#25461);
#6010=VERTEX_POINT('',#25533);
#6011=VERTEX_POINT('',#25540);
#6012=VERTEX_POINT('',#25549);
#6013=VERTEX_POINT('',#25551);
#6014=VERTEX_POINT('',#25591);
#6015=VERTEX_POINT('',#25593);
#6016=VERTEX_POINT('',#25647);
#6017=VERTEX_POINT('',#25651);
#6018=VERTEX_POINT('',#25653);
#6019=VERTEX_POINT('',#25707);
#6020=VERTEX_POINT('',#25735);
#6021=VERTEX_POINT('',#25810);
#6022=VERTEX_POINT('',#25885);
#6023=VERTEX_POINT('',#25894);
#7481=EDGE_CURVE('',#5976,#5977,#256,.T.);
#7482=EDGE_CURVE('',#5978,#5977,#257,.T.);
#7483=EDGE_CURVE('',#5978,#5979,#258,.T.);
#7484=EDGE_CURVE('',#5979,#5976,#3315,.T.);
#7485=EDGE_CURVE('',#5980,#5981,#259,.T.);
#7486=EDGE_CURVE('',#5982,#5981,#260,.T.);
#7487=EDGE_CURVE('',#5982,#5983,#261,.T.);
#7488=EDGE_CURVE('',#5983,#5980,#3316,.T.);
#7489=EDGE_CURVE('',#5981,#5984,#262,.T.);
#7490=EDGE_CURVE('',#5984,#5985,#3317,.T.);
#7491=EDGE_CURVE('',#5985,#5982,#263,.T.);
#7492=EDGE_CURVE('',#5984,#5986,#3318,.T.);
#7493=EDGE_CURVE('',#5986,#5987,#3319,.T.);
#7494=EDGE_CURVE('',#5987,#5985,#3320,.T.);
#7495=EDGE_CURVE('',#5977,#5987,#264,.T.);
#7496=EDGE_CURVE('',#5986,#5978,#265,.T.);
#7497=EDGE_CURVE('',#5988,#5979,#3321,.T.);
#7498=EDGE_CURVE('',#5989,#5988,#3322,.T.);
#7499=EDGE_CURVE('',#5990,#5989,#3323,.T.);
#7500=EDGE_CURVE('',#5991,#5990,#3324,.T.);
#7501=EDGE_CURVE('',#5992,#5991,#3325,.T.);
#7502=EDGE_CURVE('',#5993,#5992,#3326,.T.);
#7503=EDGE_CURVE('',#5976,#5993,#3327,.T.);
#7504=EDGE_CURVE('',#5986,#5994,#3328,.T.);
#7505=EDGE_CURVE('',#5995,#5994,#266,.T.);
#7506=EDGE_CURVE('',#5988,#5995,#267,.T.);
#7507=EDGE_CURVE('',#5996,#5984,#3329,.T.);
#7508=EDGE_CURVE('',#5994,#5996,#3330,.T.);
#7509=EDGE_CURVE('',#5980,#5997,#3331,.T.);
#7510=EDGE_CURVE('',#5998,#5997,#268,.T.);
#7511=EDGE_CURVE('',#5996,#5998,#269,.T.);
#7512=EDGE_CURVE('',#5999,#6000,#270,.T.);
#7513=EDGE_CURVE('',#5998,#6000,#271,.T.);
#7514=EDGE_CURVE('',#5997,#5999,#3332,.T.);
#7515=EDGE_CURVE('',#6001,#5995,#272,.T.);
#7516=EDGE_CURVE('',#6001,#5989,#273,.T.);
#7517=EDGE_CURVE('',#5994,#6002,#3333,.T.);
#7518=EDGE_CURVE('',#6002,#6001,#274,.T.);
#7519=EDGE_CURVE('',#5996,#6003,#3334,.T.);
#7520=EDGE_CURVE('',#6003,#6002,#3335,.T.);
#7521=EDGE_CURVE('',#6000,#6003,#275,.T.);
#7522=EDGE_CURVE('',#5990,#6004,#276,.T.);
#7523=EDGE_CURVE('',#6005,#6004,#277,.T.);
#7524=EDGE_CURVE('',#6005,#5991,#278,.T.);
#7525=EDGE_CURVE('',#6006,#6007,#279,.T.);
#7526=EDGE_CURVE('',#6008,#6007,#280,.T.);
#7527=EDGE_CURVE('',#6008,#6009,#281,.T.);
#7528=EDGE_CURVE('',#6009,#6006,#3336,.T.);
#7529=EDGE_CURVE('',#6007,#6010,#282,.T.);
#7530=EDGE_CURVE('',#6010,#6011,#3337,.T.);
#7531=EDGE_CURVE('',#6011,#6008,#283,.T.);
#7532=EDGE_CURVE('',#6010,#6012,#3338,.T.);
#7533=EDGE_CURVE('',#6012,#6013,#3339,.T.);
#7534=EDGE_CURVE('',#6013,#6011,#3340,.T.);
#7535=EDGE_CURVE('',#6004,#6013,#284,.T.);
#7536=EDGE_CURVE('',#6012,#6005,#285,.T.);
#7537=EDGE_CURVE('',#6012,#6014,#3341,.T.);
#7538=EDGE_CURVE('',#6015,#6014,#286,.T.);
#7539=EDGE_CURVE('',#5992,#6015,#287,.T.);
#7540=EDGE_CURVE('',#6016,#6010,#3342,.T.);
#7541=EDGE_CURVE('',#6014,#6016,#3343,.T.);
#7542=EDGE_CURVE('',#6006,#6017,#3344,.T.);
#7543=EDGE_CURVE('',#6018,#6017,#288,.T.);
#7544=EDGE_CURVE('',#6016,#6018,#289,.T.);
#7545=EDGE_CURVE('',#6019,#5983,#3345,.T.);
#7546=EDGE_CURVE('',#6017,#6019,#3346,.T.);
#7547=EDGE_CURVE('',#5999,#6009,#3347,.T.);
#7548=EDGE_CURVE('',#6020,#6015,#290,.T.);
#7549=EDGE_CURVE('',#6020,#5993,#291,.T.);
#7550=EDGE_CURVE('',#6019,#6021,#292,.T.);
#7551=EDGE_CURVE('',#6018,#6021,#293,.T.);
#7552=EDGE_CURVE('',#6021,#6022,#294,.T.);
#7553=EDGE_CURVE('',#6022,#6016,#3348,.T.);
#7554=EDGE_CURVE('',#6022,#6023,#3349,.T.);
#7555=EDGE_CURVE('',#6023,#6014,#3350,.T.);
#7556=EDGE_CURVE('',#6023,#6020,#295,.T.);
#7557=EDGE_CURVE('',#6023,#5987,#3351,.T.);
#7558=EDGE_CURVE('',#5985,#6022,#3352,.T.);
#7559=EDGE_CURVE('',#6011,#6003,#3353,.T.);
#7560=EDGE_CURVE('',#6002,#6013,#3354,.T.);
#10209=ORIENTED_EDGE('',*,*,#7481,.T.);
#10210=ORIENTED_EDGE('',*,*,#7482,.F.);
#10211=ORIENTED_EDGE('',*,*,#7483,.T.);
#10212=ORIENTED_EDGE('',*,*,#7484,.T.);
#10213=ORIENTED_EDGE('',*,*,#7485,.T.);
#10214=ORIENTED_EDGE('',*,*,#7486,.F.);
#10215=ORIENTED_EDGE('',*,*,#7487,.T.);
#10216=ORIENTED_EDGE('',*,*,#7488,.T.);
#10217=ORIENTED_EDGE('',*,*,#7486,.T.);
#10218=ORIENTED_EDGE('',*,*,#7489,.T.);
#10219=ORIENTED_EDGE('',*,*,#7490,.T.);
#10220=ORIENTED_EDGE('',*,*,#7491,.T.);
#10221=ORIENTED_EDGE('',*,*,#7490,.F.);
#10222=ORIENTED_EDGE('',*,*,#7492,.T.);
#10223=ORIENTED_EDGE('',*,*,#7493,.T.);
#10224=ORIENTED_EDGE('',*,*,#7494,.T.);
#10225=ORIENTED_EDGE('',*,*,#7482,.T.);
#10226=ORIENTED_EDGE('',*,*,#7495,.T.);
#10227=ORIENTED_EDGE('',*,*,#7493,.F.);
#10228=ORIENTED_EDGE('',*,*,#7496,.T.);
#10229=ORIENTED_EDGE('',*,*,#7484,.F.);
#10230=ORIENTED_EDGE('',*,*,#7497,.F.);
#10231=ORIENTED_EDGE('',*,*,#7498,.F.);
#10232=ORIENTED_EDGE('',*,*,#7499,.F.);
#10233=ORIENTED_EDGE('',*,*,#7500,.F.);
#10234=ORIENTED_EDGE('',*,*,#7501,.F.);
#10235=ORIENTED_EDGE('',*,*,#7502,.F.);
#10236=ORIENTED_EDGE('',*,*,#7503,.F.);
#10237=ORIENTED_EDGE('',*,*,#7483,.F.);
#10238=ORIENTED_EDGE('',*,*,#7496,.F.);
#10239=ORIENTED_EDGE('',*,*,#7504,.T.);
#10240=ORIENTED_EDGE('',*,*,#7505,.F.);
#10241=ORIENTED_EDGE('',*,*,#7506,.F.);
#10242=ORIENTED_EDGE('',*,*,#7497,.T.);
#10243=ORIENTED_EDGE('',*,*,#7492,.F.);
#10244=ORIENTED_EDGE('',*,*,#7507,.F.);
#10245=ORIENTED_EDGE('',*,*,#7508,.F.);
#10246=ORIENTED_EDGE('',*,*,#7504,.F.);
#10247=ORIENTED_EDGE('',*,*,#7489,.F.);
#10248=ORIENTED_EDGE('',*,*,#7485,.F.);
#10249=ORIENTED_EDGE('',*,*,#7509,.T.);
#10250=ORIENTED_EDGE('',*,*,#7510,.F.);
#10251=ORIENTED_EDGE('',*,*,#7511,.F.);
#10252=ORIENTED_EDGE('',*,*,#7507,.T.);
#10253=ORIENTED_EDGE('',*,*,#7512,.T.);
#10254=ORIENTED_EDGE('',*,*,#7513,.F.);
#10255=ORIENTED_EDGE('',*,*,#7510,.T.);
#10256=ORIENTED_EDGE('',*,*,#7514,.T.);
#10257=ORIENTED_EDGE('',*,*,#7506,.T.);
#10258=ORIENTED_EDGE('',*,*,#7515,.F.);
#10259=ORIENTED_EDGE('',*,*,#7516,.T.);
#10260=ORIENTED_EDGE('',*,*,#7498,.T.);
#10261=ORIENTED_EDGE('',*,*,#7515,.T.);
#10262=ORIENTED_EDGE('',*,*,#7505,.T.);
#10263=ORIENTED_EDGE('',*,*,#7517,.T.);
#10264=ORIENTED_EDGE('',*,*,#7518,.T.);
#10265=ORIENTED_EDGE('',*,*,#7519,.T.);
#10266=ORIENTED_EDGE('',*,*,#7520,.T.);
#10267=ORIENTED_EDGE('',*,*,#7517,.F.);
#10268=ORIENTED_EDGE('',*,*,#7508,.T.);
#10269=ORIENTED_EDGE('',*,*,#7513,.T.);
#10270=ORIENTED_EDGE('',*,*,#7521,.T.);
#10271=ORIENTED_EDGE('',*,*,#7519,.F.);
#10272=ORIENTED_EDGE('',*,*,#7511,.T.);
#10273=ORIENTED_EDGE('',*,*,#7522,.T.);
#10274=ORIENTED_EDGE('',*,*,#7523,.F.);
#10275=ORIENTED_EDGE('',*,*,#7524,.T.);
#10276=ORIENTED_EDGE('',*,*,#7500,.T.);
#10277=ORIENTED_EDGE('',*,*,#7525,.T.);
#10278=ORIENTED_EDGE('',*,*,#7526,.F.);
#10279=ORIENTED_EDGE('',*,*,#7527,.T.);
#10280=ORIENTED_EDGE('',*,*,#7528,.T.);
#10281=ORIENTED_EDGE('',*,*,#7526,.T.);
#10282=ORIENTED_EDGE('',*,*,#7529,.T.);
#10283=ORIENTED_EDGE('',*,*,#7530,.T.);
#10284=ORIENTED_EDGE('',*,*,#7531,.T.);
#10285=ORIENTED_EDGE('',*,*,#7530,.F.);
#10286=ORIENTED_EDGE('',*,*,#7532,.T.);
#10287=ORIENTED_EDGE('',*,*,#7533,.T.);
#10288=ORIENTED_EDGE('',*,*,#7534,.T.);
#10289=ORIENTED_EDGE('',*,*,#7523,.T.);
#10290=ORIENTED_EDGE('',*,*,#7535,.T.);
#10291=ORIENTED_EDGE('',*,*,#7533,.F.);
#10292=ORIENTED_EDGE('',*,*,#7536,.T.);
#10293=ORIENTED_EDGE('',*,*,#7524,.F.);
#10294=ORIENTED_EDGE('',*,*,#7536,.F.);
#10295=ORIENTED_EDGE('',*,*,#7537,.T.);
#10296=ORIENTED_EDGE('',*,*,#7538,.F.);
#10297=ORIENTED_EDGE('',*,*,#7539,.F.);
#10298=ORIENTED_EDGE('',*,*,#7501,.T.);
#10299=ORIENTED_EDGE('',*,*,#7532,.F.);
#10300=ORIENTED_EDGE('',*,*,#7540,.F.);
#10301=ORIENTED_EDGE('',*,*,#7541,.F.);
#10302=ORIENTED_EDGE('',*,*,#7537,.F.);
#10303=ORIENTED_EDGE('',*,*,#7529,.F.);
#10304=ORIENTED_EDGE('',*,*,#7525,.F.);
#10305=ORIENTED_EDGE('',*,*,#7542,.T.);
#10306=ORIENTED_EDGE('',*,*,#7543,.F.);
#10307=ORIENTED_EDGE('',*,*,#7544,.F.);
#10308=ORIENTED_EDGE('',*,*,#7540,.T.);
#10309=ORIENTED_EDGE('',*,*,#7488,.F.);
#10310=ORIENTED_EDGE('',*,*,#7545,.F.);
#10311=ORIENTED_EDGE('',*,*,#7546,.F.);
#10312=ORIENTED_EDGE('',*,*,#7542,.F.);
#10313=ORIENTED_EDGE('',*,*,#7528,.F.);
#10314=ORIENTED_EDGE('',*,*,#7547,.F.);
#10315=ORIENTED_EDGE('',*,*,#7514,.F.);
#10316=ORIENTED_EDGE('',*,*,#7509,.F.);
#10317=ORIENTED_EDGE('',*,*,#7539,.T.);
#10318=ORIENTED_EDGE('',*,*,#7548,.F.);
#10319=ORIENTED_EDGE('',*,*,#7549,.T.);
#10320=ORIENTED_EDGE('',*,*,#7502,.T.);
#10321=ORIENTED_EDGE('',*,*,#7550,.T.);
#10322=ORIENTED_EDGE('',*,*,#7551,.F.);
#10323=ORIENTED_EDGE('',*,*,#7543,.T.);
#10324=ORIENTED_EDGE('',*,*,#7546,.T.);
#10325=ORIENTED_EDGE('',*,*,#7551,.T.);
#10326=ORIENTED_EDGE('',*,*,#7552,.T.);
#10327=ORIENTED_EDGE('',*,*,#7553,.T.);
#10328=ORIENTED_EDGE('',*,*,#7544,.T.);
#10329=ORIENTED_EDGE('',*,*,#7553,.F.);
#10330=ORIENTED_EDGE('',*,*,#7554,.T.);
#10331=ORIENTED_EDGE('',*,*,#7555,.T.);
#10332=ORIENTED_EDGE('',*,*,#7541,.T.);
#10333=ORIENTED_EDGE('',*,*,#7548,.T.);
#10334=ORIENTED_EDGE('',*,*,#7538,.T.);
#10335=ORIENTED_EDGE('',*,*,#7555,.F.);
#10336=ORIENTED_EDGE('',*,*,#7556,.T.);
#10337=ORIENTED_EDGE('',*,*,#7481,.F.);
#10338=ORIENTED_EDGE('',*,*,#7503,.T.);
#10339=ORIENTED_EDGE('',*,*,#7549,.F.);
#10340=ORIENTED_EDGE('',*,*,#7556,.F.);
#10341=ORIENTED_EDGE('',*,*,#7557,.T.);
#10342=ORIENTED_EDGE('',*,*,#7495,.F.);
#10343=ORIENTED_EDGE('',*,*,#7494,.F.);
#10344=ORIENTED_EDGE('',*,*,#7557,.F.);
#10345=ORIENTED_EDGE('',*,*,#7554,.F.);
#10346=ORIENTED_EDGE('',*,*,#7558,.F.);
#10347=ORIENTED_EDGE('',*,*,#7491,.F.);
#10348=ORIENTED_EDGE('',*,*,#7558,.T.);
#10349=ORIENTED_EDGE('',*,*,#7552,.F.);
#10350=ORIENTED_EDGE('',*,*,#7550,.F.);
#10351=ORIENTED_EDGE('',*,*,#7545,.T.);
#10352=ORIENTED_EDGE('',*,*,#7487,.F.);
#10353=ORIENTED_EDGE('',*,*,#7512,.F.);
#10354=ORIENTED_EDGE('',*,*,#7547,.T.);
#10355=ORIENTED_EDGE('',*,*,#7527,.F.);
#10356=ORIENTED_EDGE('',*,*,#7531,.F.);
#10357=ORIENTED_EDGE('',*,*,#7559,.T.);
#10358=ORIENTED_EDGE('',*,*,#7521,.F.);
#10359=ORIENTED_EDGE('',*,*,#7520,.F.);
#10360=ORIENTED_EDGE('',*,*,#7559,.F.);
#10361=ORIENTED_EDGE('',*,*,#7534,.F.);
#10362=ORIENTED_EDGE('',*,*,#7560,.F.);
#10363=ORIENTED_EDGE('',*,*,#7518,.F.);
#10364=ORIENTED_EDGE('',*,*,#7560,.T.);
#10365=ORIENTED_EDGE('',*,*,#7535,.F.);
#10366=ORIENTED_EDGE('',*,*,#7522,.F.);
#10367=ORIENTED_EDGE('',*,*,#7499,.T.);
#10368=ORIENTED_EDGE('',*,*,#7516,.F.);
#12705=PLANE('',#14414);
#12706=PLANE('',#14415);
#12707=PLANE('',#14417);
#12708=PLANE('',#14419);
#12709=PLANE('',#14420);
#12710=PLANE('',#14422);
#12711=PLANE('',#14424);
#12712=PLANE('',#14425);
#12713=PLANE('',#14427);
#12714=PLANE('',#14430);
#13324=ADVANCED_FACE('',(#1561),#471,.T.);
#13325=ADVANCED_FACE('',(#1562),#472,.T.);
#13326=ADVANCED_FACE('',(#1563),#473,.T.);
#13327=ADVANCED_FACE('',(#1564),#12705,.T.);
#13328=ADVANCED_FACE('',(#1565),#474,.T.);
#13329=ADVANCED_FACE('',(#1566),#12706,.F.);
#13330=ADVANCED_FACE('',(#1567),#718,.T.);
#13331=ADVANCED_FACE('',(#1568),#12707,.T.);
#13332=ADVANCED_FACE('',(#1569),#719,.T.);
#13333=ADVANCED_FACE('',(#1570),#475,.T.);
#13334=ADVANCED_FACE('',(#1571),#476,.T.);
#13335=ADVANCED_FACE('',(#1572),#477,.T.);
#13336=ADVANCED_FACE('',(#1573),#12708,.T.);
#13337=ADVANCED_FACE('',(#1574),#478,.T.);
#13338=ADVANCED_FACE('',(#1575),#479,.T.);
#13339=ADVANCED_FACE('',(#1576),#480,.T.);
#13340=ADVANCED_FACE('',(#1577),#481,.T.);
#13341=ADVANCED_FACE('',(#1578),#12709,.T.);
#13342=ADVANCED_FACE('',(#1579),#482,.T.);
#13343=ADVANCED_FACE('',(#1580),#720,.T.);
#13344=ADVANCED_FACE('',(#1581),#12710,.T.);
#13345=ADVANCED_FACE('',(#1582),#721,.T.);
#13346=ADVANCED_FACE('',(#1583),#12711,.T.);
#13347=ADVANCED_FACE('',(#1584),#483,.T.);
#13348=ADVANCED_FACE('',(#1585),#484,.T.);
#13349=ADVANCED_FACE('',(#1586),#485,.T.);
#13350=ADVANCED_FACE('',(#1587),#12712,.T.);
#13351=ADVANCED_FACE('',(#1588),#486,.T.);
#13352=ADVANCED_FACE('',(#1589),#722,.T.);
#13353=ADVANCED_FACE('',(#1590),#12713,.T.);
#13354=ADVANCED_FACE('',(#1591),#723,.T.);
#13355=ADVANCED_FACE('',(#1592),#724,.T.);
#13356=ADVANCED_FACE('',(#1593),#12714,.T.);
#13357=ADVANCED_FACE('',(#1594),#725,.T.);
#13810=CLOSED_SHELL('',(#13324,#13325,#13326,#13327,#13328,#13329,#13330,
#13331,#13332,#13333,#13334,#13335,#13336,#13337,#13338,#13339,#13340,#13341,
#13342,#13343,#13344,#13345,#13346,#13347,#13348,#13349,#13350,#13351,#13352,
#13353,#13354,#13355,#13356,#13357));
#14413=AXIS2_PLACEMENT_3D('',#24576,#16303,#16304);
#14414=AXIS2_PLACEMENT_3D('',#24866,#16308,#16309);
#14415=AXIS2_PLACEMENT_3D('',#24914,#16313,#16314);
#14416=AXIS2_PLACEMENT_3D('',#24928,#16322,#16323);
#14417=AXIS2_PLACEMENT_3D('',#24984,#16325,#16326);
#14418=AXIS2_PLACEMENT_3D('',#24988,#16329,#16330);
#14419=AXIS2_PLACEMENT_3D('',#25228,#16334,#16335);
#14420=AXIS2_PLACEMENT_3D('',#25548,#16340,#16341);
#14421=AXIS2_PLACEMENT_3D('',#25590,#16345,#16346);
#14422=AXIS2_PLACEMENT_3D('',#25646,#16348,#16349);
#14423=AXIS2_PLACEMENT_3D('',#25650,#16352,#16353);
#14424=AXIS2_PLACEMENT_3D('',#25706,#16355,#16356);
#14425=AXIS2_PLACEMENT_3D('',#25893,#16361,#16362);
#14426=AXIS2_PLACEMENT_3D('',#25927,#16365,#16366);
#14427=AXIS2_PLACEMENT_3D('',#25929,#16368,#16369);
#14428=AXIS2_PLACEMENT_3D('',#25931,#16371,#16372);
#14429=AXIS2_PLACEMENT_3D('',#25932,#16373,#16374);
#14430=AXIS2_PLACEMENT_3D('',#25934,#16376,#16377);
#14431=AXIS2_PLACEMENT_3D('',#25936,#16379,#16380);
#16303=DIRECTION('axis',(0.,0.,1.));
#16304=DIRECTION('refdir',(1.,0.,0.));
#16305=DIRECTION('',(0.707106781186503,0.,0.707106781186592));
#16306=DIRECTION('',(-0.707106781186503,0.,-0.707106781186592));
#16307=DIRECTION('',(0.707106781186563,0.,0.707106781186532));
#16308=DIRECTION('center_axis',(-0.707106781186548,0.,0.707106781186548));
#16309=DIRECTION('ref_axis',(0.707106781186548,0.,0.707106781186548));
#16310=DIRECTION('',(0.,-1.,0.));
#16311=DIRECTION('',(0.707106781186563,0.,0.707106781186532));
#16312=DIRECTION('',(0.,1.,0.));
#16313=DIRECTION('center_axis',(0.,1.,0.));
#16314=DIRECTION('ref_axis',(1.,0.,0.));
#16315=DIRECTION('',(0.,0.,1.));
#16316=DIRECTION('',(-0.70710678118657,0.,0.707106781186525));
#16317=DIRECTION('',(-1.,0.,0.));
#16318=DIRECTION('',(-0.707106781186556,0.,-0.707106781186539));
#16319=DIRECTION('',(0.,0.,-1.));
#16320=DIRECTION('',(0.707106781186545,0.,-0.70710678118655));
#16321=DIRECTION('',(1.,0.,0.));
#16322=DIRECTION('center_axis',(0.,0.,-1.));
#16323=DIRECTION('ref_axis',(-0.707106781186555,-0.70710678118654,0.));
#16324=DIRECTION('',(0.,0.,-1.));
#16325=DIRECTION('center_axis',(-1.,0.,0.));
#16326=DIRECTION('ref_axis',(0.,0.,1.));
#16327=DIRECTION('',(0.,0.,1.));
#16328=DIRECTION('',(0.,1.,0.));
#16329=DIRECTION('center_axis',(0.,0.,1.));
#16330=DIRECTION('ref_axis',(-0.707106781186555,0.70710678118654,0.));
#16331=DIRECTION('',(0.,0.,-1.));
#16332=DIRECTION('',(0.70710678118657,0.,-0.707106781186525));
#16333=DIRECTION('',(0.707106781186548,0.,-0.707106781186548));
#16334=DIRECTION('center_axis',(-0.707106781186548,0.,-0.707106781186548));
#16335=DIRECTION('ref_axis',(-0.707106781186548,0.,0.707106781186548));
#16336=DIRECTION('',(0.707106781186548,0.,-0.707106781186548));
#16337=DIRECTION('',(0.,-1.,0.));
#16338=DIRECTION('',(0.707106781186511,0.,0.707106781186584));
#16339=DIRECTION('',(-0.707106781186563,0.,-0.707106781186532));
#16340=DIRECTION('center_axis',(0.707106781186538,0.,-0.707106781186557));
#16341=DIRECTION('ref_axis',(-0.707106781186557,0.,-0.707106781186538));
#16342=DIRECTION('',(0.,-1.,0.));
#16343=DIRECTION('',(-0.707106781186557,0.,-0.707106781186538));
#16344=DIRECTION('',(0.,1.,0.));
#16345=DIRECTION('center_axis',(0.,0.,1.));
#16346=DIRECTION('ref_axis',(0.707106781186555,-0.70710678118654,0.));
#16347=DIRECTION('',(0.,0.,1.));
#16348=DIRECTION('center_axis',(1.,0.,0.));
#16349=DIRECTION('ref_axis',(0.,0.,-1.));
#16350=DIRECTION('',(0.,0.,-1.));
#16351=DIRECTION('',(0.,1.,0.));
#16352=DIRECTION('center_axis',(0.,0.,-1.));
#16353=DIRECTION('ref_axis',(0.707106781186555,0.70710678118654,0.));
#16354=DIRECTION('',(0.,0.,1.));
#16355=DIRECTION('center_axis',(0.,1.,0.));
#16356=DIRECTION('ref_axis',(0.,0.,1.));
#16357=DIRECTION('',(-1.,0.,0.));
#16358=DIRECTION('',(-0.707106781186534,0.,0.707106781186561));
#16359=DIRECTION('',(1.,0.,0.));
#16360=DIRECTION('',(0.707106781186575,0.,-0.70710678118652));
#16361=DIRECTION('center_axis',(0.707106781186538,0.,0.707106781186557));
#16362=DIRECTION('ref_axis',(0.707106781186557,0.,-0.707106781186538));
#16363=DIRECTION('',(0.,-1.,0.));
#16364=DIRECTION('',(0.707106781186557,0.,-0.707106781186538));
#16365=DIRECTION('center_axis',(-1.,0.,0.));
#16366=DIRECTION('ref_axis',(0.,-0.70710678118654,0.707106781186555));
#16367=DIRECTION('',(-1.,0.,0.));
#16368=DIRECTION('center_axis',(0.,0.,1.));
#16369=DIRECTION('ref_axis',(1.,0.,0.));
#16370=DIRECTION('',(1.,0.,0.));
#16371=DIRECTION('center_axis',(1.,0.,0.));
#16372=DIRECTION('ref_axis',(0.,0.70710678118654,0.707106781186555));
#16373=DIRECTION('center_axis',(-1.,0.,0.));
#16374=DIRECTION('ref_axis',(0.,0.707106781186532,-0.707106781186563));
#16375=DIRECTION('',(-1.,0.,0.));
#16376=DIRECTION('center_axis',(0.,0.,-1.));
#16377=DIRECTION('ref_axis',(-1.,0.,0.));
#16378=DIRECTION('',(1.,0.,0.));
#16379=DIRECTION('center_axis',(1.,0.,0.));
#16380=DIRECTION('ref_axis',(0.,-0.707106781186532,-0.707106781186563));
#24576=CARTESIAN_POINT('',(0.,0.,0.));
#24577=CARTESIAN_POINT('Ctrl Pts',(-66.2975371703006,122.238070190751,43.6801990080023));
#24578=CARTESIAN_POINT('Ctrl Pts',(-66.295869694655,122.238006634921,43.678516554556));
#24579=CARTESIAN_POINT('Ctrl Pts',(-66.2836640413214,122.237567815036,43.6661713539299));
#24580=CARTESIAN_POINT('Ctrl Pts',(-66.2702842984222,122.237504067589,43.6526075471718));
#24581=CARTESIAN_POINT('Ctrl Pts',(-66.2681224083043,122.2375,43.6504214071384));
#24582=CARTESIAN_POINT('Ctrl Pts',(-66.2677059397486,122.2375,43.65));
#24583=CARTESIAN_POINT('Ctrl Pts',(-66.3917577828678,122.238070190751,43.5859783954351));
#24584=CARTESIAN_POINT('Ctrl Pts',(-66.390085314622,122.238006634921,43.584300934589));
#24585=CARTESIAN_POINT('Ctrl Pts',(-66.3778263299278,122.237567815036,43.5720090653235));
#24586=CARTESIAN_POINT('Ctrl Pts',(-66.3643944630001,122.237504067589,43.558497382594));
#24587=CARTESIAN_POINT('Ctrl Pts',(-66.3622220745824,122.2375,43.5563217408604));
#24588=CARTESIAN_POINT('Ctrl Pts',(-66.3618039598324,122.2375,43.5559019799162));
#24589=CARTESIAN_POINT('Ctrl Pts',(-66.4859783954351,122.238070190751,43.4917577828678));
#24590=CARTESIAN_POINT('Ctrl Pts',(-66.484300934589,122.238006634921,43.490085314622));
#24591=CARTESIAN_POINT('Ctrl Pts',(-66.4719682708158,122.237492703884,43.4778263299279));
#24592=CARTESIAN_POINT('Ctrl Pts',(-66.4584917270448,122.23754961255,43.464394463));
#24593=CARTESIAN_POINT('Ctrl Pts',(-66.4563217408604,122.2375,43.4622220745823));
#24594=CARTESIAN_POINT('Ctrl Pts',(-66.4559019799162,122.2375,43.4618039598323));
#24595=CARTESIAN_POINT('Ctrl Pts',(-66.5801990080023,122.238070190751,43.3975371703006));
#24596=CARTESIAN_POINT('Ctrl Pts',(-66.578516554556,122.238006634921,43.395869694655));
#24597=CARTESIAN_POINT('Ctrl Pts',(-66.5661713539299,122.237567815036,43.3836640413215));
#24598=CARTESIAN_POINT('Ctrl Pts',(-66.5526075471718,122.237504067589,43.3702842984222));
#24599=CARTESIAN_POINT('Ctrl Pts',(-66.5504214071384,122.2375,43.3681224083043));
#24600=CARTESIAN_POINT('Ctrl Pts',(-66.55,122.2375,43.3677059397485));
#24601=CARTESIAN_POINT('',(-66.2677059397486,122.2375,43.65));
#24602=CARTESIAN_POINT('',(-66.2975371703006,122.238070190751,43.6801990080023));
#24603=CARTESIAN_POINT('Ctrl Pts',(-66.2677059397486,122.2375,43.65));
#24604=CARTESIAN_POINT('Ctrl Pts',(-66.2678726988052,122.2375,43.650168736525));
#24605=CARTESIAN_POINT('Ctrl Pts',(-66.2680426727623,122.237500039141,43.6503407294752));
#24606=CARTESIAN_POINT('Ctrl Pts',(-66.2682711198522,122.237500204467,43.6505719684178));
#24607=CARTESIAN_POINT('Ctrl Pts',(-66.2685232393849,122.237500386926,43.6508271691041));
#24608=CARTESIAN_POINT('Ctrl Pts',(-66.2688465074852,122.23750071898,43.6511544591101));
#24609=CARTESIAN_POINT('Ctrl Pts',(-66.2692682628933,122.237501563317,43.6515815512717));
#24610=CARTESIAN_POINT('Ctrl Pts',(-66.2697392792016,122.237502506272,43.6520585276647));
#24611=CARTESIAN_POINT('Ctrl Pts',(-66.2703326618206,122.237504104656,43.6526595049514));
#24612=CARTESIAN_POINT('Ctrl Pts',(-66.2710345962128,122.237507100231,43.6533705073353));
#24613=CARTESIAN_POINT('Ctrl Pts',(-66.271922356591,122.237510888837,43.6542697363121));
#24614=CARTESIAN_POINT('Ctrl Pts',(-66.2729823430601,122.237517016609,43.6553435322326));
#24615=CARTESIAN_POINT('Ctrl Pts',(-66.274119373636,122.237526369906,43.6564954718404));
#24616=CARTESIAN_POINT('Ctrl Pts',(-66.275267024347,122.237535810566,43.6576581708371));
#24617=CARTESIAN_POINT('Ctrl Pts',(-66.2764877640867,122.237548536479,43.6588950097937));
#24618=CARTESIAN_POINT('Ctrl Pts',(-66.2776823234139,122.237563826519,43.6601053627627));
#24619=CARTESIAN_POINT('Ctrl Pts',(-66.2785768692241,122.237575276466,43.6610117356425));
#24620=CARTESIAN_POINT('Ctrl Pts',(-66.2794562057464,122.237588088159,43.6619027203554));
#24621=CARTESIAN_POINT('Ctrl Pts',(-66.2803059516487,122.237601826337,43.6627636895375));
#24622=CARTESIAN_POINT('Ctrl Pts',(-66.2810774585305,122.237614299594,43.6635453863334));
#24623=CARTESIAN_POINT('Ctrl Pts',(-66.2818241823993,122.237627497267,43.6643019452828));
#24624=CARTESIAN_POINT('Ctrl Pts',(-66.2825668820939,122.237641657879,43.6650543196431));
#24625=CARTESIAN_POINT('Ctrl Pts',(-66.2833438316762,122.237656471514,43.6658413900423));
#24626=CARTESIAN_POINT('Ctrl Pts',(-66.2841235557123,122.23767247258,43.6666311424701));
#24627=CARTESIAN_POINT('Ctrl Pts',(-66.2849308055329,122.237690305677,43.6674485777765));
#24628=CARTESIAN_POINT('Ctrl Pts',(-66.2858320241453,122.237710214654,43.6683611675274));
#24629=CARTESIAN_POINT('Ctrl Pts',(-66.286766994243,122.237732447118,43.6693076969554));
#24630=CARTESIAN_POINT('Ctrl Pts',(-66.2877173601371,122.237756826022,43.6702695751379));
#24631=CARTESIAN_POINT('Ctrl Pts',(-66.2889597634694,122.237788696307,43.6715270283639));
#24632=CARTESIAN_POINT('Ctrl Pts',(-66.2902267818597,122.237824333785,43.6728089911267));
#24633=CARTESIAN_POINT('Ctrl Pts',(-66.2914048119203,122.237860099073,43.6740006009414));
#24634=CARTESIAN_POINT('Ctrl Pts',(-66.2923675692485,122.237889328627,43.6749744564649));
#24635=CARTESIAN_POINT('Ctrl Pts',(-66.293267661289,122.237918483816,43.6758847018469));
#24636=CARTESIAN_POINT('Ctrl Pts',(-66.2940452683694,122.237944709538,43.6766709110186));
#24637=CARTESIAN_POINT('Ctrl Pts',(-66.2947223806606,122.237967545954,43.6773555137016));
#24638=CARTESIAN_POINT('Ctrl Pts',(-66.2953057241463,122.237988087761,43.6779451634303));
#24639=CARTESIAN_POINT('Ctrl Pts',(-66.295779966785,122.238005126535,43.6784244138564));
#24640=CARTESIAN_POINT('Ctrl Pts',(-66.2962183038067,122.238020875278,43.6788673795184));
#24641=CARTESIAN_POINT('Ctrl Pts',(-66.2965629424176,122.238033598544,43.679215532934));
#24642=CARTESIAN_POINT('Ctrl Pts',(-66.2968329073597,122.238043654136,43.6794881511418));
#24643=CARTESIAN_POINT('Ctrl Pts',(-66.2970837268897,122.238052996604,43.6797414357728));
#24644=CARTESIAN_POINT('Ctrl Pts',(-66.297269873309,122.238060029675,43.6799293013871));
#24645=CARTESIAN_POINT('Ctrl Pts',(-66.297439207674,122.238066462969,43.6801001639575));
#24646=CARTESIAN_POINT('Ctrl Pts',(-66.2974722152538,122.238067716982,43.6801334694236));
#24647=CARTESIAN_POINT('Ctrl Pts',(-66.2975046952455,122.238068952964,43.6801662412459));
#24648=CARTESIAN_POINT('Ctrl Pts',(-66.2975371703006,122.238070190751,43.6801990080023));
#24649=CARTESIAN_POINT('',(-66.5801990080023,122.238070190751,43.3975371703006));
#24650=CARTESIAN_POINT('Ctrl Pts',(-66.5801990080023,122.238070190751,43.3975371703006));
#24651=CARTESIAN_POINT('Ctrl Pts',(-66.4859783954351,122.238070190751,43.4917577828678));
#24652=CARTESIAN_POINT('Ctrl Pts',(-66.3917577828678,122.238070190751,43.5859783954351));
#24653=CARTESIAN_POINT('Ctrl Pts',(-66.2975371703006,122.238070190751,43.6801990080023));
#24654=CARTESIAN_POINT('',(-66.55,122.2375,43.3677059397485));
#24655=CARTESIAN_POINT('Ctrl Pts',(-66.5801990080023,122.238070190751,43.3975371703006));
#24656=CARTESIAN_POINT('Ctrl Pts',(-66.5800305855052,122.238063828476,43.3973702471606));
#24657=CARTESIAN_POINT('Ctrl Pts',(-66.5798589093858,122.238057382362,43.397200107149));
#24658=CARTESIAN_POINT('Ctrl Pts',(-66.579628057339,122.23804882687,43.3969714633112));
#24659=CARTESIAN_POINT('Ctrl Pts',(-66.579373282892,122.238039384803,43.3967191259023));
#24660=CARTESIAN_POINT('Ctrl Pts',(-66.579046504163,122.238027372131,43.3963956021263));
#24661=CARTESIAN_POINT('Ctrl Pts',(-66.5786200261656,122.238012105093,43.3959735434092));
#24662=CARTESIAN_POINT('Ctrl Pts',(-66.5781437326004,122.237995054761,43.3955021853267));
#24663=CARTESIAN_POINT('Ctrl Pts',(-66.5775435637608,122.237973979824,43.3949084001561));
#24664=CARTESIAN_POINT('Ctrl Pts',(-66.5768334404113,122.237950147598,43.3942060222412));
#24665=CARTESIAN_POINT('Ctrl Pts',(-66.5759352908255,122.237920005083,43.3933176689237));
#24666=CARTESIAN_POINT('Ctrl Pts',(-66.5748626695,122.237885609635,43.3922570121513));
#24667=CARTESIAN_POINT('Ctrl Pts',(-66.5737118227387,122.237851483799,43.3911193310077));
#24668=CARTESIAN_POINT('Ctrl Pts',(-66.5725503239299,122.2378170421,43.3899711196752));
#24669=CARTESIAN_POINT('Ctrl Pts',(-66.5713146082228,122.237783080562,43.3887498553891));
#24670=CARTESIAN_POINT('Ctrl Pts',(-66.5701051310901,122.237752675088,43.3875548864531));
#24671=CARTESIAN_POINT('Ctrl Pts',(-66.5691994017694,122.237729905638,43.3866600217438));
#24672=CARTESIAN_POINT('Ctrl Pts',(-66.5683089239631,122.237709074602,43.3857804315059));
#24673=CARTESIAN_POINT('Ctrl Pts',(-66.5674482886096,122.237690299368,43.3849305199691));
#24674=CARTESIAN_POINT('Ctrl Pts',(-66.5666668879855,122.237673252684,43.3841588558693));
#24675=CARTESIAN_POINT('Ctrl Pts',(-66.5659104838912,122.237657876347,43.3834120480763));
#24676=CARTESIAN_POINT('Ctrl Pts',(-66.5651581113835,122.237643618104,43.3826693398989));
#24677=CARTESIAN_POINT('Ctrl Pts',(-66.5643710534174,122.237628702536,43.3818923918027));
#24678=CARTESIAN_POINT('Ctrl Pts',(-66.5635811455704,122.237614869895,43.3811127516152));
#24679=CARTESIAN_POINT('Ctrl Pts',(-66.5627634000951,122.237601821718,43.3803056659794));
#24680=CARTESIAN_POINT('Ctrl Pts',(-66.5618504525924,122.237587254472,43.3794046193358));
#24681=CARTESIAN_POINT('Ctrl Pts',(-66.5609033701718,122.237573726381,43.378469920108));
#24682=CARTESIAN_POINT('Ctrl Pts',(-66.5599407885337,122.237561764432,43.377519896467));
#24683=CARTESIAN_POINT('Ctrl Pts',(-66.5586823476285,122.237546125856,43.3762778733873));
#24684=CARTESIAN_POINT('Ctrl Pts',(-66.5573991342584,122.237533328235,43.3750113535098));
#24685=CARTESIAN_POINT('Ctrl Pts',(-66.5562062234238,122.237524073618,43.3738338670347));
#24686=CARTESIAN_POINT('Ctrl Pts',(-66.555231427366,122.237516511138,43.3728716751083));
#24687=CARTESIAN_POINT('Ctrl Pts',(-66.5543201973287,122.237511277906,43.3719721616152));
#24688=CARTESIAN_POINT('Ctrl Pts',(-66.5535330697621,122.237507801652,43.3711950841759));
#24689=CARTESIAN_POINT('Ctrl Pts',(-66.5528476493566,122.237504774575,43.37051841529));
#24690=CARTESIAN_POINT('Ctrl Pts',(-66.5522572394504,122.237503040519,43.3699354824523));
#24691=CARTESIAN_POINT('Ctrl Pts',(-66.5517773349746,122.237501974327,43.3694615957548));
#24692=CARTESIAN_POINT('Ctrl Pts',(-66.5513337613121,122.237500988851,43.369023584299));
#24693=CARTESIAN_POINT('Ctrl Pts',(-66.5509850931076,122.237500559908,43.3686792256942));
#24694=CARTESIAN_POINT('Ctrl Pts',(-66.5507120440952,122.237500316879,43.3684094978756));
#24695=CARTESIAN_POINT('Ctrl Pts',(-66.5504583577137,122.237500091084,43.3681588971731));
#24696=CARTESIAN_POINT('Ctrl Pts',(-66.5502701637948,122.237500027304,43.3679729332267));
#24697=CARTESIAN_POINT('Ctrl Pts',(-66.5500989877785,122.237500006124,43.3678037667746));
#24698=CARTESIAN_POINT('Ctrl Pts',(-66.5500656344477,122.237500001997,43.3677708050036));
#24699=CARTESIAN_POINT('Ctrl Pts',(-66.5500328147292,122.2375,43.3677383699132));
#24700=CARTESIAN_POINT('Ctrl Pts',(-66.55,122.2375,43.3677059397485));
#24701=CARTESIAN_POINT('',(-66.4088529698743,122.2375,43.5088529698743));
#24702=CARTESIAN_POINT('Ctrl Pts',(-66.5801990080023,126.999429809249,43.3975371703006));
#24703=CARTESIAN_POINT('Ctrl Pts',(-66.578516554556,126.999493365079,43.395869694655));
#24704=CARTESIAN_POINT('Ctrl Pts',(-66.5661715453635,126.999932181252,43.383664231718));
#24705=CARTESIAN_POINT('Ctrl Pts',(-66.5526075968239,126.999995931781,43.3702843477267));
#24706=CARTESIAN_POINT('Ctrl Pts',(-66.5504214071384,127.,43.3681224083043));
#24707=CARTESIAN_POINT('Ctrl Pts',(-66.55,127.,43.3677059397485));
#24708=CARTESIAN_POINT('Ctrl Pts',(-66.4859783954351,126.999429809249,43.4917577828678));
#24709=CARTESIAN_POINT('Ctrl Pts',(-66.484300934589,126.999493365079,43.490085314622));
#24710=CARTESIAN_POINT('Ctrl Pts',(-66.4720092567571,126.999932181252,43.4778265203243));
#24711=CARTESIAN_POINT('Ctrl Pts',(-66.458497432246,126.999995931781,43.4643945123045));
#24712=CARTESIAN_POINT('Ctrl Pts',(-66.4563217408604,127.,43.4622220745824));
#24713=CARTESIAN_POINT('Ctrl Pts',(-66.4559019799162,127.,43.4618039598323));
#24714=CARTESIAN_POINT('Ctrl Pts',(-66.3917577828678,126.999429809249,43.5859783954351));
#24715=CARTESIAN_POINT('Ctrl Pts',(-66.390085314622,126.999493365079,43.584300934589));
#24716=CARTESIAN_POINT('Ctrl Pts',(-66.3778265203244,127.000007314886,43.5719684631258));
#24717=CARTESIAN_POINT('Ctrl Pts',(-66.3643945123046,126.999950392654,43.5584917768456));
#24718=CARTESIAN_POINT('Ctrl Pts',(-66.3622220745824,127.,43.5563217408604));
#24719=CARTESIAN_POINT('Ctrl Pts',(-66.3618039598324,127.,43.5559019799162));
#24720=CARTESIAN_POINT('Ctrl Pts',(-66.2975371703006,126.999429809249,43.6801990080023));
#24721=CARTESIAN_POINT('Ctrl Pts',(-66.295869694655,126.999493365079,43.678516554556));
#24722=CARTESIAN_POINT('Ctrl Pts',(-66.283664231718,126.999932181252,43.6661715453635));
#24723=CARTESIAN_POINT('Ctrl Pts',(-66.2702843477267,126.999995931781,43.6526075968239));
#24724=CARTESIAN_POINT('Ctrl Pts',(-66.2681224083043,127.,43.6504214071384));
#24725=CARTESIAN_POINT('Ctrl Pts',(-66.2677059397486,127.,43.65));
#24726=CARTESIAN_POINT('',(-66.55,127.,43.3677059397485));
#24727=CARTESIAN_POINT('',(-66.5801990080023,126.999429809249,43.3975371703006));
#24728=CARTESIAN_POINT('Ctrl Pts',(-66.55,127.,43.3677059397485));
#24729=CARTESIAN_POINT('Ctrl Pts',(-66.550168736525,127.,43.3678726988052));
#24730=CARTESIAN_POINT('Ctrl Pts',(-66.5503407294752,126.999999960859,43.3680426727623));
#24731=CARTESIAN_POINT('Ctrl Pts',(-66.5505719684178,126.999999795533,43.3682711198522));
#24732=CARTESIAN_POINT('Ctrl Pts',(-66.5508271691041,126.999999613074,43.3685232393849));
#24733=CARTESIAN_POINT('Ctrl Pts',(-66.5511544591101,126.99999928102,43.3688465074852));
#24734=CARTESIAN_POINT('Ctrl Pts',(-66.5515815512717,126.999998436683,43.3692682628933));
#24735=CARTESIAN_POINT('Ctrl Pts',(-66.5520585276647,126.999997493728,43.3697392792016));
#24736=CARTESIAN_POINT('Ctrl Pts',(-66.5526595049514,126.999995895344,43.3703326618206));
#24737=CARTESIAN_POINT('Ctrl Pts',(-66.5533705073353,126.999992899769,43.3710345962128));
#24738=CARTESIAN_POINT('Ctrl Pts',(-66.554269736312,126.999989111163,43.371922356591));
#24739=CARTESIAN_POINT('Ctrl Pts',(-66.5553435322326,126.999982983391,43.37298234306));
#24740=CARTESIAN_POINT('Ctrl Pts',(-66.5564954718403,126.999973630094,43.3741193736359));
#24741=CARTESIAN_POINT('Ctrl Pts',(-66.5576581708369,126.999964189434,43.3752670243469));
#24742=CARTESIAN_POINT('Ctrl Pts',(-66.5588950097936,126.999951463521,43.3764877640866));
#24743=CARTESIAN_POINT('Ctrl Pts',(-66.5601053627626,126.999936173481,43.3776823234138));
#24744=CARTESIAN_POINT('Ctrl Pts',(-66.5610117356423,126.999924723534,43.378576869224));
#24745=CARTESIAN_POINT('Ctrl Pts',(-66.5619027203552,126.999911911841,43.3794562057463));
#24746=CARTESIAN_POINT('Ctrl Pts',(-66.5627636895374,126.999898173663,43.3803059516486));
#24747=CARTESIAN_POINT('Ctrl Pts',(-66.5635453863323,126.999885700406,43.3810774585295));
#24748=CARTESIAN_POINT('Ctrl Pts',(-66.5643019452809,126.999872502733,43.3818241823974));
#24749=CARTESIAN_POINT('Ctrl Pts',(-66.5650543196403,126.999858342121,43.3825668820911));
#24750=CARTESIAN_POINT('Ctrl Pts',(-66.5658413900395,126.999843528486,43.3833438316734));
#24751=CARTESIAN_POINT('Ctrl Pts',(-66.5666311424671,126.99982752742,43.3841235557094));
#24752=CARTESIAN_POINT('Ctrl Pts',(-66.5674485777734,126.999809694323,43.3849308055298));
#24753=CARTESIAN_POINT('Ctrl Pts',(-66.5683611675241,126.999789785346,43.385832024142));
#24754=CARTESIAN_POINT('Ctrl Pts',(-66.5693076969518,126.999767552882,43.3867669942395));
#24755=CARTESIAN_POINT('Ctrl Pts',(-66.5702695751342,126.999743173978,43.3877173601334));
#24756=CARTESIAN_POINT('Ctrl Pts',(-66.5715270283595,126.999711303693,43.3889597634651));
#24757=CARTESIAN_POINT('Ctrl Pts',(-66.5728089911216,126.999675666215,43.3902267818547));
#24758=CARTESIAN_POINT('Ctrl Pts',(-66.5740006009359,126.999639900927,43.3914048119149));
#24759=CARTESIAN_POINT('Ctrl Pts',(-66.57497445646,126.999610671373,43.3923675692436));
#24760=CARTESIAN_POINT('Ctrl Pts',(-66.5758847018426,126.999581516184,43.3932676612848));
#24761=CARTESIAN_POINT('Ctrl Pts',(-66.5766709110149,126.999555290462,43.3940452683658));
#24762=CARTESIAN_POINT('Ctrl Pts',(-66.5773555136983,126.999532454046,43.3947223806574));
#24763=CARTESIAN_POINT('Ctrl Pts',(-66.5779451634274,126.999511912239,43.3953057241435));
#24764=CARTESIAN_POINT('Ctrl Pts',(-66.5784244138539,126.999494873465,43.3957799667826));
#24765=CARTESIAN_POINT('Ctrl Pts',(-66.5788673795163,126.999479124722,43.3962183038047));
#24766=CARTESIAN_POINT('Ctrl Pts',(-66.5792155329322,126.999466401456,43.3965629424159));
#24767=CARTESIAN_POINT('Ctrl Pts',(-66.5794881511403,126.999456345864,43.3968329073583));
#24768=CARTESIAN_POINT('Ctrl Pts',(-66.5797414357716,126.999447003396,43.3970837268885));
#24769=CARTESIAN_POINT('Ctrl Pts',(-66.5799293013861,126.999439970325,43.3972698733081));
#24770=CARTESIAN_POINT('Ctrl Pts',(-66.5801001639566,126.999433537031,43.3974392076731));
#24771=CARTESIAN_POINT('Ctrl Pts',(-66.580133469423,126.999432283018,43.3974722152533));
#24772=CARTESIAN_POINT('Ctrl Pts',(-66.5801662412456,126.999431047036,43.3975046952452));
#24773=CARTESIAN_POINT('Ctrl Pts',(-66.5801990080023,126.999429809249,43.3975371703006));
#24774=CARTESIAN_POINT('',(-66.2975371703006,126.999429809249,43.6801990080023));
#24775=CARTESIAN_POINT('Ctrl Pts',(-66.2975371703006,126.999429809249,43.6801990080023));
#24776=CARTESIAN_POINT('Ctrl Pts',(-66.3917577828678,126.999429809249,43.5859783954351));
#24777=CARTESIAN_POINT('Ctrl Pts',(-66.4859783954351,126.999429809249,43.4917577828678));
#24778=CARTESIAN_POINT('Ctrl Pts',(-66.5801990080023,126.999429809249,43.3975371703006));
#24779=CARTESIAN_POINT('',(-66.2677059397486,127.,43.65));
#24780=CARTESIAN_POINT('Ctrl Pts',(-66.2975371703006,126.999429809249,43.6801990080023));
#24781=CARTESIAN_POINT('Ctrl Pts',(-66.2973702471606,126.999436171524,43.6800305855052));
#24782=CARTESIAN_POINT('Ctrl Pts',(-66.2972001071489,126.999442617638,43.6798589093858));
#24783=CARTESIAN_POINT('Ctrl Pts',(-66.296971463311,126.99945117313,43.6796280573389));
#24784=CARTESIAN_POINT('Ctrl Pts',(-66.2967191259022,126.999460615197,43.6793732828919));
#24785=CARTESIAN_POINT('Ctrl Pts',(-66.2963956021262,126.999472627869,43.6790465041628));
#24786=CARTESIAN_POINT('Ctrl Pts',(-66.295973543409,126.999487894907,43.6786200261654));
#24787=CARTESIAN_POINT('Ctrl Pts',(-66.2955021853265,126.999504945239,43.6781437326002));
#24788=CARTESIAN_POINT('Ctrl Pts',(-66.2949084001558,126.999526020176,43.6775435637606));
#24789=CARTESIAN_POINT('Ctrl Pts',(-66.2942060222409,126.999549852402,43.676833440411));
#24790=CARTESIAN_POINT('Ctrl Pts',(-66.2933176689234,126.999579994917,43.6759352908252));
#24791=CARTESIAN_POINT('Ctrl Pts',(-66.2922570121512,126.999614390365,43.6748626694998));
#24792=CARTESIAN_POINT('Ctrl Pts',(-66.2911193310076,126.999648516201,43.6737118227387));
#24793=CARTESIAN_POINT('Ctrl Pts',(-66.2899711196751,126.9996829579,43.6725503239299));
#24794=CARTESIAN_POINT('Ctrl Pts',(-66.288749855389,126.999716919438,43.6713146082227));
#24795=CARTESIAN_POINT('Ctrl Pts',(-66.287554886453,126.999747324912,43.6701051310901));
#24796=CARTESIAN_POINT('Ctrl Pts',(-66.2866600217437,126.999770094362,43.6691994017693));
#24797=CARTESIAN_POINT('Ctrl Pts',(-66.2857804315058,126.999790925398,43.668308923963));
#24798=CARTESIAN_POINT('Ctrl Pts',(-66.284930519969,126.999809700632,43.6674482886095));
#24799=CARTESIAN_POINT('Ctrl Pts',(-66.2841588558683,126.999826747316,43.6666668879845));
#24800=CARTESIAN_POINT('Ctrl Pts',(-66.2834120480745,126.999842123653,43.6659104838894));
#24801=CARTESIAN_POINT('Ctrl Pts',(-66.2826693398963,126.999856381896,43.6651581113809));
#24802=CARTESIAN_POINT('Ctrl Pts',(-66.2818923918,126.999871297464,43.6643710534147));
#24803=CARTESIAN_POINT('Ctrl Pts',(-66.2811127516125,126.999885130105,43.6635811455676));
#24804=CARTESIAN_POINT('Ctrl Pts',(-66.2803056659765,126.999898178282,43.6627634000922));
#24805=CARTESIAN_POINT('Ctrl Pts',(-66.2794046193328,126.999912745528,43.6618504525894));
#24806=CARTESIAN_POINT('Ctrl Pts',(-66.2784699201047,126.999926273619,43.6609033701686));
#24807=CARTESIAN_POINT('Ctrl Pts',(-66.2775198964636,126.999938235568,43.6599407885303));
#24808=CARTESIAN_POINT('Ctrl Pts',(-66.276277873383,126.999953874144,43.6586823476241));
#24809=CARTESIAN_POINT('Ctrl Pts',(-66.2750113535045,126.999966671765,43.6573991342531));
#24810=CARTESIAN_POINT('Ctrl Pts',(-66.2738338670289,126.999975926382,43.6562062234179));
#24811=CARTESIAN_POINT('Ctrl Pts',(-66.2728716751032,126.999983488862,43.6552314273608));
#24812=CARTESIAN_POINT('Ctrl Pts',(-66.2719721616108,126.999988722094,43.6543201973242));
#24813=CARTESIAN_POINT('Ctrl Pts',(-66.2711950841722,126.999992198348,43.6535330697583));
#24814=CARTESIAN_POINT('Ctrl Pts',(-66.2705184152867,126.999995225425,43.6528476493533));
#24815=CARTESIAN_POINT('Ctrl Pts',(-66.2699354824495,126.999996959481,43.6522572394475));
#24816=CARTESIAN_POINT('Ctrl Pts',(-66.2694615957523,126.999998025673,43.6517773349722));
#24817=CARTESIAN_POINT('Ctrl Pts',(-66.2690235842969,126.999999011149,43.6513337613101));
#24818=CARTESIAN_POINT('Ctrl Pts',(-66.2686792256925,126.999999440092,43.6509850931059));
#24819=CARTESIAN_POINT('Ctrl Pts',(-66.2684094978742,126.999999683121,43.6507120440938));
#24820=CARTESIAN_POINT('Ctrl Pts',(-66.268158897172,126.999999908916,43.6504583577125));
#24821=CARTESIAN_POINT('Ctrl Pts',(-66.2679729332258,126.999999972695,43.6502701637938));
#24822=CARTESIAN_POINT('Ctrl Pts',(-66.2678037667737,126.999999993876,43.6500989877776));
#24823=CARTESIAN_POINT('Ctrl Pts',(-66.267770805003,126.999999998003,43.6500656344471));
#24824=CARTESIAN_POINT('Ctrl Pts',(-66.2677383699129,127.,43.6500328147289));
#24825=CARTESIAN_POINT('Ctrl Pts',(-66.2677059397486,127.,43.65));
#24826=CARTESIAN_POINT('',(-66.4088529698743,127.,43.5088529698743));
#24827=CARTESIAN_POINT('Ctrl Pts',(-66.2975371703006,126.999429809249,43.6801990080023));
#24828=CARTESIAN_POINT('Ctrl Pts',(-66.4934491246469,126.991962625601,43.8778707063143));
#24829=CARTESIAN_POINT('Ctrl Pts',(-66.8258588963354,126.852169790253,44.1891309474517));
#24830=CARTESIAN_POINT('Ctrl Pts',(-67.1039178520905,126.497789859875,44.4167876971285));
#24831=CARTESIAN_POINT('Ctrl Pts',(-67.15,126.297687701072,44.45));
#24832=CARTESIAN_POINT('Ctrl Pts',(-67.15,126.2,44.45));
#24833=CARTESIAN_POINT('Ctrl Pts',(-66.3917577828678,126.999429809249,43.5859783954351));
#24834=CARTESIAN_POINT('Ctrl Pts',(-66.5882563185361,126.991962625601,43.7830635124252));
#24835=CARTESIAN_POINT('Ctrl Pts',(-66.9136162467075,126.852169790253,44.1013735970796));
#24836=CARTESIAN_POINT('Ctrl Pts',(-67.1748744671032,126.497789859875,44.3458310821159));
#24837=CARTESIAN_POINT('Ctrl Pts',(-67.2166666666667,126.297687701072,44.3833333333333));
#24838=CARTESIAN_POINT('Ctrl Pts',(-67.2166666666667,126.2,44.3833333333333));
#24839=CARTESIAN_POINT('Ctrl Pts',(-66.4859783954351,126.999429809249,43.4917577828678));
#24840=CARTESIAN_POINT('Ctrl Pts',(-66.6830635124252,126.991962625601,43.6882563185361));
#24841=CARTESIAN_POINT('Ctrl Pts',(-67.0013735970796,126.852169790253,44.0136162467075));
#24842=CARTESIAN_POINT('Ctrl Pts',(-67.2458310821159,126.497789859875,44.2748744671032));
#24843=CARTESIAN_POINT('Ctrl Pts',(-67.2833333333333,126.297687701072,44.3166666666667));
#24844=CARTESIAN_POINT('Ctrl Pts',(-67.2833333333333,126.2,44.3166666666667));
#24845=CARTESIAN_POINT('Ctrl Pts',(-66.5801990080023,126.999429809249,43.3975371703006));
#24846=CARTESIAN_POINT('Ctrl Pts',(-66.7778707063143,126.991962625601,43.5934491246469));
#24847=CARTESIAN_POINT('Ctrl Pts',(-67.0891309474517,126.852169790253,43.9258588963354));
#24848=CARTESIAN_POINT('Ctrl Pts',(-67.3167876971285,126.497789859875,44.2039178520906));
#24849=CARTESIAN_POINT('Ctrl Pts',(-67.35,126.297687701072,44.25));
#24850=CARTESIAN_POINT('Ctrl Pts',(-67.35,126.2,44.25));
#24851=CARTESIAN_POINT('',(-67.35,126.2,44.25));
#24852=CARTESIAN_POINT('Ctrl Pts',(-66.5801990080023,126.999429809249,43.3975371703006));
#24853=CARTESIAN_POINT('Ctrl Pts',(-66.7778707063143,126.991962625601,43.5934491246469));
#24854=CARTESIAN_POINT('Ctrl Pts',(-67.0891309474517,126.852169790253,43.9258588963354));
#24855=CARTESIAN_POINT('Ctrl Pts',(-67.3167876971285,126.497789859875,44.2039178520906));
#24856=CARTESIAN_POINT('Ctrl Pts',(-67.35,126.297687701072,44.25));
#24857=CARTESIAN_POINT('Ctrl Pts',(-67.35,126.2,44.25));
#24858=CARTESIAN_POINT('',(-67.15,126.2,44.45));
#24859=CARTESIAN_POINT('',(-67.35,126.2,44.25));
#24860=CARTESIAN_POINT('Ctrl Pts',(-67.15,126.2,44.45));
#24861=CARTESIAN_POINT('Ctrl Pts',(-67.15,126.297687701072,44.45));
#24862=CARTESIAN_POINT('Ctrl Pts',(-67.1039178520905,126.497789859875,44.4167876971285));
#24863=CARTESIAN_POINT('Ctrl Pts',(-66.8258588963354,126.852169790253,44.1891309474517));
#24864=CARTESIAN_POINT('Ctrl Pts',(-66.4934491246469,126.991962625601,43.8778707063143));
#24865=CARTESIAN_POINT('Ctrl Pts',(-66.2975371703006,126.999429809249,43.6801990080023));
#24866=CARTESIAN_POINT('Origin',(-67.25,122.2375,44.35));
#24867=CARTESIAN_POINT('',(-67.35,123.0375,44.25));
#24868=CARTESIAN_POINT('',(-67.35,122.2375,44.25));
#24869=CARTESIAN_POINT('',(-67.15,123.0375,44.45));
#24870=CARTESIAN_POINT('',(-67.35,123.0375,44.25));
#24871=CARTESIAN_POINT('',(-67.15,122.2375,44.45));
#24872=CARTESIAN_POINT('Ctrl Pts',(-67.15,123.0375,44.45));
#24873=CARTESIAN_POINT('Ctrl Pts',(-67.15,122.964234224196,44.45));
#24874=CARTESIAN_POINT('Ctrl Pts',(-67.124110265378,122.816497863585,44.4310410082707));
#24875=CARTESIAN_POINT('Ctrl Pts',(-66.979153924583,122.559479514224,44.3164595240405));
#24876=CARTESIAN_POINT('Ctrl Pts',(-66.6927364773364,122.319066835802,44.066950725335));
#24877=CARTESIAN_POINT('Ctrl Pts',(-66.4281451398648,122.243048313183,43.8119801402103));
#24878=CARTESIAN_POINT('Ctrl Pts',(-66.2975371703006,122.238070190751,43.6801990080023));
#24879=CARTESIAN_POINT('Ctrl Pts',(-67.2166666666667,123.0375,44.3833333333333));
#24880=CARTESIAN_POINT('Ctrl Pts',(-67.2166666666667,122.964234224196,44.3833333333333));
#24881=CARTESIAN_POINT('Ctrl Pts',(-67.1930871796756,122.816497863585,44.3620640939731));
#24882=CARTESIAN_POINT('Ctrl Pts',(-67.0582557910688,122.559479514224,44.2373576575547));
#24883=CARTESIAN_POINT('Ctrl Pts',(-66.7841412266692,122.319066835802,43.9755459760021));
#24884=CARTESIAN_POINT('Ctrl Pts',(-66.5227568066466,122.243048313183,43.7173684734285));
#24885=CARTESIAN_POINT('Ctrl Pts',(-66.3917577828678,122.238070190751,43.5859783954351));
#24886=CARTESIAN_POINT('Ctrl Pts',(-67.2833333333333,123.0375,44.3166666666667));
#24887=CARTESIAN_POINT('Ctrl Pts',(-67.2833333333333,122.964234224196,44.3166666666667));
#24888=CARTESIAN_POINT('Ctrl Pts',(-67.2620640939731,122.816497863585,44.2930871796756));
#24889=CARTESIAN_POINT('Ctrl Pts',(-67.1373576575547,122.559479514224,44.1582557910688));
#24890=CARTESIAN_POINT('Ctrl Pts',(-66.8755459760021,122.319066835802,43.8841412266693));
#24891=CARTESIAN_POINT('Ctrl Pts',(-66.6173684734285,122.243048313183,43.6227568066467));
#24892=CARTESIAN_POINT('Ctrl Pts',(-66.4859783954351,122.238070190751,43.4917577828678));
#24893=CARTESIAN_POINT('Ctrl Pts',(-67.35,123.0375,44.25));
#24894=CARTESIAN_POINT('Ctrl Pts',(-67.35,122.964234224196,44.25));
#24895=CARTESIAN_POINT('Ctrl Pts',(-67.3310410082707,122.816497863585,44.224110265378));
#24896=CARTESIAN_POINT('Ctrl Pts',(-67.2164595240405,122.559479514224,44.079153924583));
#24897=CARTESIAN_POINT('Ctrl Pts',(-66.966950725335,122.319066835802,43.7927364773364));
#24898=CARTESIAN_POINT('Ctrl Pts',(-66.7119801402103,122.243048313183,43.5281451398648));
#24899=CARTESIAN_POINT('Ctrl Pts',(-66.5801990080023,122.238070190751,43.3975371703006));
#24900=CARTESIAN_POINT('Ctrl Pts',(-66.2975371703006,122.238070190751,43.6801990080023));
#24901=CARTESIAN_POINT('Ctrl Pts',(-66.4281451398648,122.243048313183,43.8119801402103));
#24902=CARTESIAN_POINT('Ctrl Pts',(-66.6927364773364,122.319066835802,44.066950725335));
#24903=CARTESIAN_POINT('Ctrl Pts',(-66.979153924583,122.559479514224,44.3164595240405));
#24904=CARTESIAN_POINT('Ctrl Pts',(-67.124110265378,122.816497863585,44.4310410082707));
#24905=CARTESIAN_POINT('Ctrl Pts',(-67.15,122.964234224196,44.45));
#24906=CARTESIAN_POINT('Ctrl Pts',(-67.15,123.0375,44.45));
#24907=CARTESIAN_POINT('Ctrl Pts',(-67.35,123.0375,44.25));
#24908=CARTESIAN_POINT('Ctrl Pts',(-67.35,122.964234224196,44.25));
#24909=CARTESIAN_POINT('Ctrl Pts',(-67.3310410082707,122.816497863585,44.224110265378));
#24910=CARTESIAN_POINT('Ctrl Pts',(-67.2164595240405,122.559479514224,44.079153924583));
#24911=CARTESIAN_POINT('Ctrl Pts',(-66.966950725335,122.319066835802,43.7927364773364));
#24912=CARTESIAN_POINT('Ctrl Pts',(-66.7119801402103,122.243048313183,43.5281451398648));
#24913=CARTESIAN_POINT('Ctrl Pts',(-66.5801990080023,122.238070190751,43.3975371703006));
#24914=CARTESIAN_POINT('Origin',(-29.25,122.2375,-31.75));
#24915=CARTESIAN_POINT('',(-66.55,122.2375,-106.867705939749));
#24916=CARTESIAN_POINT('',(-66.55,122.2375,-69.85));
#24917=CARTESIAN_POINT('',(-66.2677059397485,122.2375,-107.15));
#24918=CARTESIAN_POINT('',(-66.4088529698743,122.2375,-107.008852969874));
#24919=CARTESIAN_POINT('',(7.76770593974857,122.2375,-107.15));
#24920=CARTESIAN_POINT('',(-10.2,122.2375,-107.15));
#24921=CARTESIAN_POINT('',(8.05,122.2375,-106.867705939749));
#24922=CARTESIAN_POINT('',(7.90885296987428,122.2375,-107.008852969874));
#24923=CARTESIAN_POINT('',(8.05,122.2375,43.3677059397486));
#24924=CARTESIAN_POINT('',(8.05,122.2375,6.35000000000001));
#24925=CARTESIAN_POINT('',(7.76770593974856,122.2375,43.65));
#24926=CARTESIAN_POINT('',(7.90885296987428,122.2375,43.5088529698743));
#24927=CARTESIAN_POINT('',(-48.3,122.2375,43.65));
#24928=CARTESIAN_POINT('Origin',(-66.55,123.0375,-69.85));
#24929=CARTESIAN_POINT('',(-67.35,123.0375,-107.75));
#24930=CARTESIAN_POINT('',(-67.35,123.0375,-69.85));
#24931=CARTESIAN_POINT('',(-66.5801990080023,122.238070190751,-106.897537170301));
#24932=CARTESIAN_POINT('Ctrl Pts',(-66.5801990080023,122.238070190751,-106.897537170301));
#24933=CARTESIAN_POINT('Ctrl Pts',(-66.7778707063143,122.245537374399,-107.093449124647));
#24934=CARTESIAN_POINT('Ctrl Pts',(-67.0891343165395,122.385328730462,-107.425865391595));
#24935=CARTESIAN_POINT('Ctrl Pts',(-67.3167943482721,122.739701425857,-107.703924410673));
#24936=CARTESIAN_POINT('Ctrl Pts',(-67.35,122.939812298928,-107.75));
#24937=CARTESIAN_POINT('Ctrl Pts',(-67.35,123.0375,-107.75));
#24938=CARTESIAN_POINT('Ctrl Pts',(-66.55,122.2375,-106.867705939749));
#24939=CARTESIAN_POINT('Ctrl Pts',(-66.550168736525,122.2375,-106.867872698805));
#24940=CARTESIAN_POINT('Ctrl Pts',(-66.5503407294752,122.237500039141,-106.868042672762));
#24941=CARTESIAN_POINT('Ctrl Pts',(-66.5505719684178,122.237500204467,-106.868271119852));
#24942=CARTESIAN_POINT('Ctrl Pts',(-66.5508271691041,122.237500386926,-106.868523239385));
#24943=CARTESIAN_POINT('Ctrl Pts',(-66.5511544591101,122.23750071898,-106.868846507485));
#24944=CARTESIAN_POINT('Ctrl Pts',(-66.5515815512717,122.237501563317,-106.869268262893));
#24945=CARTESIAN_POINT('Ctrl Pts',(-66.5520585276647,122.237502506272,-106.869739279202));
#24946=CARTESIAN_POINT('Ctrl Pts',(-66.5526595049514,122.237504104656,-106.870332661821));
#24947=CARTESIAN_POINT('Ctrl Pts',(-66.5533705073353,122.237507100231,-106.871034596213));
#24948=CARTESIAN_POINT('Ctrl Pts',(-66.5542697363121,122.237510888837,-106.871922356591));
#24949=CARTESIAN_POINT('Ctrl Pts',(-66.5553435322327,122.237517016609,-106.87298234306));
#24950=CARTESIAN_POINT('Ctrl Pts',(-66.5564954718406,122.237526369906,-106.874119373636));
#24951=CARTESIAN_POINT('Ctrl Pts',(-66.5576581708372,122.237535810566,-106.875267024347));
#24952=CARTESIAN_POINT('Ctrl Pts',(-66.5588950097939,122.237548536479,-106.876487764087));
#24953=CARTESIAN_POINT('Ctrl Pts',(-66.5601053627629,122.237563826519,-106.877682323414));
#24954=CARTESIAN_POINT('Ctrl Pts',(-66.5610117356426,122.237575276466,-106.878576869224));
#24955=CARTESIAN_POINT('Ctrl Pts',(-66.5619027203555,122.237588088159,-106.879456205747));
#24956=CARTESIAN_POINT('Ctrl Pts',(-66.5627636895377,122.237601826337,-106.880305951649));
#24957=CARTESIAN_POINT('Ctrl Pts',(-66.5635453863286,122.237614299594,-106.881077458526));
#24958=CARTESIAN_POINT('Ctrl Pts',(-66.5643019452735,122.237627497267,-106.88182418239));
#24959=CARTESIAN_POINT('Ctrl Pts',(-66.5650543196291,122.237641657879,-106.88256688208));
#24960=CARTESIAN_POINT('Ctrl Pts',(-66.565841390028,122.237656471514,-106.883343831662));
#24961=CARTESIAN_POINT('Ctrl Pts',(-66.5666311424552,122.23767247258,-106.884123555698));
#24962=CARTESIAN_POINT('Ctrl Pts',(-66.567448577761,122.237690305676,-106.884930805518));
#24963=CARTESIAN_POINT('Ctrl Pts',(-66.5683611675107,122.237710214654,-106.885832024129));
#24964=CARTESIAN_POINT('Ctrl Pts',(-66.5693076969374,122.237732447118,-106.886766994225));
#24965=CARTESIAN_POINT('Ctrl Pts',(-66.570269575119,122.237756826022,-106.887717360118));
#24966=CARTESIAN_POINT('Ctrl Pts',(-66.5715270283396,122.237788696306,-106.888959763445));
#24967=CARTESIAN_POINT('Ctrl Pts',(-66.5728089910973,122.237824333784,-106.890226781831));
#24968=CARTESIAN_POINT('Ctrl Pts',(-66.5740006009088,122.237860099072,-106.891404811888));
#24969=CARTESIAN_POINT('Ctrl Pts',(-66.5749744564358,122.237889328626,-106.89236756922));
#24970=CARTESIAN_POINT('Ctrl Pts',(-66.5758847018216,122.237918483815,-106.893267661264));
#24971=CARTESIAN_POINT('Ctrl Pts',(-66.5766709109972,122.237944709537,-106.894045268348));
#24972=CARTESIAN_POINT('Ctrl Pts',(-66.5773555136828,122.237967545954,-106.894722380642));
#24973=CARTESIAN_POINT('Ctrl Pts',(-66.5779451634142,122.23798808776,-106.89530572413));
#24974=CARTESIAN_POINT('Ctrl Pts',(-66.5784244138428,122.238005126534,-106.895779966772));
#24975=CARTESIAN_POINT('Ctrl Pts',(-66.578867379507,122.238020875277,-106.896218303795));
#24976=CARTESIAN_POINT('Ctrl Pts',(-66.5792155329245,122.238033598544,-106.896562942408));
#24977=CARTESIAN_POINT('Ctrl Pts',(-66.5794881511339,122.238043654136,-106.896832907352));
#24978=CARTESIAN_POINT('Ctrl Pts',(-66.5797414357662,122.238052996604,-106.897083726883));
#24979=CARTESIAN_POINT('Ctrl Pts',(-66.5799293013816,122.238060029674,-106.897269873304));
#24980=CARTESIAN_POINT('Ctrl Pts',(-66.5801001639524,122.238066462969,-106.897439207669));
#24981=CARTESIAN_POINT('Ctrl Pts',(-66.5801334694202,122.238067716982,-106.89747221525));
#24982=CARTESIAN_POINT('Ctrl Pts',(-66.5801662412442,122.238068952964,-106.897504695244));
#24983=CARTESIAN_POINT('Ctrl Pts',(-66.5801990080023,122.238070190751,-106.897537170301));
#24984=CARTESIAN_POINT('Origin',(-67.35,122.2375,-107.95));
#24985=CARTESIAN_POINT('',(-67.35,126.2,-107.75));
#24986=CARTESIAN_POINT('',(-67.35,126.2,-69.85));
#24987=CARTESIAN_POINT('',(-67.35,122.2375,-107.75));
#24988=CARTESIAN_POINT('Origin',(-66.55,126.2,-69.85));
#24989=CARTESIAN_POINT('',(-66.55,127.,-106.867705939749));
#24990=CARTESIAN_POINT('',(-66.55,127.,-69.85));
#24991=CARTESIAN_POINT('',(-66.5801990080024,126.999429809249,-106.897537170301));
#24992=CARTESIAN_POINT('Ctrl Pts',(-66.5801990080024,126.999429809249,-106.897537170301));
#24993=CARTESIAN_POINT('Ctrl Pts',(-66.5800305855052,126.999436171524,-106.897370247161));
#24994=CARTESIAN_POINT('Ctrl Pts',(-66.5798589093858,126.999442617638,-106.897200107149));
#24995=CARTESIAN_POINT('Ctrl Pts',(-66.5796280573389,126.99945117313,-106.896971463311));
#24996=CARTESIAN_POINT('Ctrl Pts',(-66.5793732828919,126.999460615197,-106.896719125902));
#24997=CARTESIAN_POINT('Ctrl Pts',(-66.5790465041629,126.999472627869,-106.896395602126));
#24998=CARTESIAN_POINT('Ctrl Pts',(-66.5786200261654,126.999487894907,-106.895973543409));
#24999=CARTESIAN_POINT('Ctrl Pts',(-66.5781437326002,126.999504945239,-106.895502185326));
#25000=CARTESIAN_POINT('Ctrl Pts',(-66.5775435637605,126.999526020176,-106.894908400156));
#25001=CARTESIAN_POINT('Ctrl Pts',(-66.576833440411,126.999549852402,-106.894206022241));
#25002=CARTESIAN_POINT('Ctrl Pts',(-66.5759352908252,126.999579994917,-106.893317668923));
#25003=CARTESIAN_POINT('Ctrl Pts',(-66.5748626694997,126.999614390365,-106.892257012151));
#25004=CARTESIAN_POINT('Ctrl Pts',(-66.5737118227385,126.999648516201,-106.891119331007));
#25005=CARTESIAN_POINT('Ctrl Pts',(-66.5725503239297,126.9996829579,-106.889971119675));
#25006=CARTESIAN_POINT('Ctrl Pts',(-66.5713146082226,126.999716919438,-106.888749855389));
#25007=CARTESIAN_POINT('Ctrl Pts',(-66.5701051310899,126.999747324912,-106.887554886453));
#25008=CARTESIAN_POINT('Ctrl Pts',(-66.5691994017692,126.999770094362,-106.886660021744));
#25009=CARTESIAN_POINT('Ctrl Pts',(-66.5683089239628,126.999790925398,-106.885780431506));
#25010=CARTESIAN_POINT('Ctrl Pts',(-66.5674482886093,126.999809700632,-106.884930519969));
#25011=CARTESIAN_POINT('Ctrl Pts',(-66.5666668879872,126.999826747316,-106.884158855871));
#25012=CARTESIAN_POINT('Ctrl Pts',(-66.5659104838949,126.999842123653,-106.88341204808));
#25013=CARTESIAN_POINT('Ctrl Pts',(-66.5651581113891,126.999856381896,-106.882669339904));
#25014=CARTESIAN_POINT('Ctrl Pts',(-66.5643710534231,126.999871297464,-106.881892391808));
#25015=CARTESIAN_POINT('Ctrl Pts',(-66.5635811455763,126.999885130105,-106.881112751621));
#25016=CARTESIAN_POINT('Ctrl Pts',(-66.5627634001013,126.999898178281,-106.880305665985));
#25017=CARTESIAN_POINT('Ctrl Pts',(-66.5618504525991,126.999912745528,-106.879404619342));
#25018=CARTESIAN_POINT('Ctrl Pts',(-66.5609033701791,126.999926273619,-106.878469920115));
#25019=CARTESIAN_POINT('Ctrl Pts',(-66.5599407885413,126.999938235568,-106.877519896475));
#25020=CARTESIAN_POINT('Ctrl Pts',(-66.5586823476381,126.999953874144,-106.876277873397));
#25021=CARTESIAN_POINT('Ctrl Pts',(-66.55739913427,126.999966671765,-106.875011353521));
#25022=CARTESIAN_POINT('Ctrl Pts',(-66.5562062234366,126.999975926382,-106.873833867047));
#25023=CARTESIAN_POINT('Ctrl Pts',(-66.5552314273775,126.999983488862,-106.87287167512));
#25024=CARTESIAN_POINT('Ctrl Pts',(-66.5543201973387,126.999988722094,-106.871972161625));
#25025=CARTESIAN_POINT('Ctrl Pts',(-66.5535330697706,126.999992198348,-106.871195084184));
#25026=CARTESIAN_POINT('Ctrl Pts',(-66.552847649364,126.999995225425,-106.870518415297));
#25027=CARTESIAN_POINT('Ctrl Pts',(-66.5522572394567,126.999996959481,-106.869935482459));
#25028=CARTESIAN_POINT('Ctrl Pts',(-66.5517773349799,126.999998025673,-106.86946159576));
#25029=CARTESIAN_POINT('Ctrl Pts',(-66.5513337613166,126.999999011149,-106.869023584303));
#25030=CARTESIAN_POINT('Ctrl Pts',(-66.5509850931112,126.999999440092,-106.868679225698));
#25031=CARTESIAN_POINT('Ctrl Pts',(-66.5507120440982,126.999999683121,-106.868409497879));
#25032=CARTESIAN_POINT('Ctrl Pts',(-66.5504583577162,126.999999908916,-106.868158897176));
#25033=CARTESIAN_POINT('Ctrl Pts',(-66.5502701637969,126.999999972695,-106.867972933229));
#25034=CARTESIAN_POINT('Ctrl Pts',(-66.5500989877805,126.999999993876,-106.867803766777));
#25035=CARTESIAN_POINT('Ctrl Pts',(-66.550065634449,126.999999998003,-106.867770805005));
#25036=CARTESIAN_POINT('Ctrl Pts',(-66.5500328147298,127.,-106.867738369914));
#25037=CARTESIAN_POINT('Ctrl Pts',(-66.55,127.,-106.867705939749));
#25038=CARTESIAN_POINT('Ctrl Pts',(-67.35,126.2,-107.75));
#25039=CARTESIAN_POINT('Ctrl Pts',(-67.35,126.297687701072,-107.75));
#25040=CARTESIAN_POINT('Ctrl Pts',(-67.3167946468525,126.497798963876,-107.703924706682));
#25041=CARTESIAN_POINT('Ctrl Pts',(-67.0891344719334,126.852171342114,-107.425865686481));
#25042=CARTESIAN_POINT('Ctrl Pts',(-66.7778707063143,126.991962625601,-107.093449124647));
#25043=CARTESIAN_POINT('Ctrl Pts',(-66.5801990080024,126.999429809249,-106.897537170301));
#25044=CARTESIAN_POINT('Ctrl Pts',(-66.2975371703006,126.999429809249,-107.180199008002));
#25045=CARTESIAN_POINT('Ctrl Pts',(-66.295869694655,126.999493365079,-107.178516554556));
#25046=CARTESIAN_POINT('Ctrl Pts',(-66.2836662133258,126.999932142639,-107.16617353777));
#25047=CARTESIAN_POINT('Ctrl Pts',(-66.270284862015,126.999995925185,-107.152608114732));
#25048=CARTESIAN_POINT('Ctrl Pts',(-66.2681224083043,127.,-107.150421407138));
#25049=CARTESIAN_POINT('Ctrl Pts',(-66.2677059397485,127.,-107.15));
#25050=CARTESIAN_POINT('Ctrl Pts',(-66.3917577828678,126.999429809249,-107.085978395435));
#25051=CARTESIAN_POINT('Ctrl Pts',(-66.390085314622,126.999493365079,-107.084300934589));
#25052=CARTESIAN_POINT('Ctrl Pts',(-66.3778285019322,126.999932142639,-107.072011249164));
#25053=CARTESIAN_POINT('Ctrl Pts',(-66.3643950265928,126.999995925185,-107.058497950154));
#25054=CARTESIAN_POINT('Ctrl Pts',(-66.3622220745824,127.,-107.05632174086));
#25055=CARTESIAN_POINT('Ctrl Pts',(-66.3618039598324,127.,-107.055901979916));
#25056=CARTESIAN_POINT('Ctrl Pts',(-66.4859783954351,126.999429809249,-106.991757782868));
#25057=CARTESIAN_POINT('Ctrl Pts',(-66.484300934589,126.999493365079,-106.990085314622));
#25058=CARTESIAN_POINT('Ctrl Pts',(-66.4719704646475,127.000007510264,-106.977828501932));
#25059=CARTESIAN_POINT('Ctrl Pts',(-66.4584922963115,126.999950446903,-106.964395026593));
#25060=CARTESIAN_POINT('Ctrl Pts',(-66.4563217408604,127.,-106.962222074582));
#25061=CARTESIAN_POINT('Ctrl Pts',(-66.4559019799162,127.,-106.961803959832));
#25062=CARTESIAN_POINT('Ctrl Pts',(-66.5801990080024,126.999429809249,-106.897537170301));
#25063=CARTESIAN_POINT('Ctrl Pts',(-66.578516554556,126.999493365079,-106.895869694655));
#25064=CARTESIAN_POINT('Ctrl Pts',(-66.5661735377701,126.999932142639,-106.883666213326));
#25065=CARTESIAN_POINT('Ctrl Pts',(-66.5526081147318,126.999995925185,-106.870284862015));
#25066=CARTESIAN_POINT('Ctrl Pts',(-66.5504214071384,127.,-106.868122408304));
#25067=CARTESIAN_POINT('Ctrl Pts',(-66.55,127.,-106.867705939749));
#25068=CARTESIAN_POINT('',(-66.2677059397485,127.,-107.15));
#25069=CARTESIAN_POINT('',(-66.2975371703006,126.999429809249,-107.180199008002));
#25070=CARTESIAN_POINT('Ctrl Pts',(-66.2677059397485,127.,-107.15));
#25071=CARTESIAN_POINT('Ctrl Pts',(-66.2678726988052,127.,-107.150168736525));
#25072=CARTESIAN_POINT('Ctrl Pts',(-66.2680426727622,126.999999960859,-107.150340729475));
#25073=CARTESIAN_POINT('Ctrl Pts',(-66.2682711198522,126.999999795533,-107.150571968418));
#25074=CARTESIAN_POINT('Ctrl Pts',(-66.2685232393849,126.999999613074,-107.150827169104));
#25075=CARTESIAN_POINT('Ctrl Pts',(-66.2688465074851,126.99999928102,-107.15115445911));
#25076=CARTESIAN_POINT('Ctrl Pts',(-66.2692682628932,126.999998436683,-107.151581551272));
#25077=CARTESIAN_POINT('Ctrl Pts',(-66.2697392792015,126.999997493728,-107.152058527665));
#25078=CARTESIAN_POINT('Ctrl Pts',(-66.2703326618206,126.999995895344,-107.152659504951));
#25079=CARTESIAN_POINT('Ctrl Pts',(-66.2710345962128,126.999992899769,-107.153370507335));
#25080=CARTESIAN_POINT('Ctrl Pts',(-66.2719223565911,126.999989111163,-107.154269736312));
#25081=CARTESIAN_POINT('Ctrl Pts',(-66.2729823430602,126.999982983391,-107.155343532233));
#25082=CARTESIAN_POINT('Ctrl Pts',(-66.2741193736363,126.999973630094,-107.156495471841));
#25083=CARTESIAN_POINT('Ctrl Pts',(-66.2752670243472,126.999964189434,-107.157658170837));
#25084=CARTESIAN_POINT('Ctrl Pts',(-66.276487764087,126.999951463521,-107.158895009794));
#25085=CARTESIAN_POINT('Ctrl Pts',(-66.2776823234141,126.999936173481,-107.160105362763));
#25086=CARTESIAN_POINT('Ctrl Pts',(-66.2785768692244,126.999924723534,-107.161011735643));
#25087=CARTESIAN_POINT('Ctrl Pts',(-66.2794562057467,126.999911911841,-107.161902720356));
#25088=CARTESIAN_POINT('Ctrl Pts',(-66.280305951649,126.999898173663,-107.162763689538));
#25089=CARTESIAN_POINT('Ctrl Pts',(-66.2810774585299,126.999885700406,-107.163545386333));
#25090=CARTESIAN_POINT('Ctrl Pts',(-66.2818241823979,126.999872502733,-107.164301945281));
#25091=CARTESIAN_POINT('Ctrl Pts',(-66.2825668820916,126.999858342121,-107.165054319641));
#25092=CARTESIAN_POINT('Ctrl Pts',(-66.2833438316739,126.999843528486,-107.16584139004));
#25093=CARTESIAN_POINT('Ctrl Pts',(-66.2841235557099,126.99982752742,-107.166631142468));
#25094=CARTESIAN_POINT('Ctrl Pts',(-66.2849308055304,126.999809694323,-107.167448577774));
#25095=CARTESIAN_POINT('Ctrl Pts',(-66.2858320241426,126.999789785346,-107.168361167525));
#25096=CARTESIAN_POINT('Ctrl Pts',(-66.2867669942401,126.999767552882,-107.169307696952));
#25097=CARTESIAN_POINT('Ctrl Pts',(-66.287717360134,126.999743173978,-107.170269575135));
#25098=CARTESIAN_POINT('Ctrl Pts',(-66.2889597634652,126.999711303693,-107.17152702836));
#25099=CARTESIAN_POINT('Ctrl Pts',(-66.2902267818545,126.999675666215,-107.172808991121));
#25100=CARTESIAN_POINT('Ctrl Pts',(-66.2914048119143,126.999639900927,-107.174000600935));
#25101=CARTESIAN_POINT('Ctrl Pts',(-66.2923675692431,126.999610671373,-107.174974456459));
#25102=CARTESIAN_POINT('Ctrl Pts',(-66.2932676612844,126.999581516184,-107.175884701842));
#25103=CARTESIAN_POINT('Ctrl Pts',(-66.2940452683655,126.999555290462,-107.176670911015));
#25104=CARTESIAN_POINT('Ctrl Pts',(-66.2947223806571,126.999532454046,-107.177355513698));
#25105=CARTESIAN_POINT('Ctrl Pts',(-66.2953057241434,126.999511912239,-107.177945163427));
#25106=CARTESIAN_POINT('Ctrl Pts',(-66.2957799667826,126.999494873465,-107.178424413854));
#25107=CARTESIAN_POINT('Ctrl Pts',(-66.2962183038047,126.999479124722,-107.178867379516));
#25108=CARTESIAN_POINT('Ctrl Pts',(-66.2965629424158,126.999466401456,-107.179215532932));
#25109=CARTESIAN_POINT('Ctrl Pts',(-66.2968329073583,126.999456345864,-107.17948815114));
#25110=CARTESIAN_POINT('Ctrl Pts',(-66.2970837268885,126.999447003396,-107.179741435772));
#25111=CARTESIAN_POINT('Ctrl Pts',(-66.297269873308,126.999439970325,-107.179929301386));
#25112=CARTESIAN_POINT('Ctrl Pts',(-66.297439207673,126.999433537031,-107.180100163957));
#25113=CARTESIAN_POINT('Ctrl Pts',(-66.2974722152532,126.999432283018,-107.180133469423));
#25114=CARTESIAN_POINT('Ctrl Pts',(-66.2975046952452,126.999431047036,-107.180166241246));
#25115=CARTESIAN_POINT('Ctrl Pts',(-66.2975371703006,126.999429809249,-107.180199008002));
#25116=CARTESIAN_POINT('Ctrl Pts',(-66.5801990080024,126.999429809249,-106.897537170301));
#25117=CARTESIAN_POINT('Ctrl Pts',(-66.4859783954351,126.999429809249,-106.991757782868));
#25118=CARTESIAN_POINT('Ctrl Pts',(-66.3917577828678,126.999429809249,-107.085978395435));
#25119=CARTESIAN_POINT('Ctrl Pts',(-66.2975371703006,126.999429809249,-107.180199008002));
#25120=CARTESIAN_POINT('',(-66.4088529698743,127.,-107.008852969874));
#25121=CARTESIAN_POINT('Ctrl Pts',(-66.5801990080023,122.238070190751,-106.897537170301));
#25122=CARTESIAN_POINT('Ctrl Pts',(-66.578516554556,122.238006634921,-106.895869694655));
#25123=CARTESIAN_POINT('Ctrl Pts',(-66.5661734170446,122.237567855022,-106.883666093255));
#25124=CARTESIAN_POINT('Ctrl Pts',(-66.5526080832916,122.237504074413,-106.870284830794));
#25125=CARTESIAN_POINT('Ctrl Pts',(-66.5504214071384,122.2375,-106.868122408304));
#25126=CARTESIAN_POINT('Ctrl Pts',(-66.55,122.2375,-106.867705939749));
#25127=CARTESIAN_POINT('Ctrl Pts',(-66.4859783954351,122.238070190751,-106.991757782868));
#25128=CARTESIAN_POINT('Ctrl Pts',(-66.484300934589,122.238006634921,-106.990085314622));
#25129=CARTESIAN_POINT('Ctrl Pts',(-66.4720111284382,122.237567855022,-106.977828381861));
#25130=CARTESIAN_POINT('Ctrl Pts',(-66.4584979187138,122.237504074413,-106.964394995372));
#25131=CARTESIAN_POINT('Ctrl Pts',(-66.4563217408604,122.2375,-106.962222074582));
#25132=CARTESIAN_POINT('Ctrl Pts',(-66.4559019799162,122.2375,-106.961803959832));
#25133=CARTESIAN_POINT('Ctrl Pts',(-66.3917577828678,122.238070190751,-107.085978395435));
#25134=CARTESIAN_POINT('Ctrl Pts',(-66.390085314622,122.238006634921,-107.084300934589));
#25135=CARTESIAN_POINT('Ctrl Pts',(-66.3778283818612,122.237492501576,-107.07197034337));
#25136=CARTESIAN_POINT('Ctrl Pts',(-66.3643949953721,122.237549556389,-107.058492264776));
#25137=CARTESIAN_POINT('Ctrl Pts',(-66.3622220745824,122.2375,-107.05632174086));
#25138=CARTESIAN_POINT('Ctrl Pts',(-66.3618039598324,122.2375,-107.055901979916));
#25139=CARTESIAN_POINT('Ctrl Pts',(-66.2975371703006,122.238070190751,-107.180199008002));
#25140=CARTESIAN_POINT('Ctrl Pts',(-66.295869694655,122.238006634921,-107.178516554556));
#25141=CARTESIAN_POINT('Ctrl Pts',(-66.2836660932549,122.237567855022,-107.166173417045));
#25142=CARTESIAN_POINT('Ctrl Pts',(-66.2702848307942,122.237504074413,-107.152608083292));
#25143=CARTESIAN_POINT('Ctrl Pts',(-66.2681224083043,122.2375,-107.150421407138));
#25144=CARTESIAN_POINT('Ctrl Pts',(-66.2677059397485,122.2375,-107.15));
#25145=CARTESIAN_POINT('',(-66.2975371703006,122.238070190751,-107.180199008002));
#25146=CARTESIAN_POINT('Ctrl Pts',(-66.2975371703006,122.238070190751,-107.180199008002));
#25147=CARTESIAN_POINT('Ctrl Pts',(-66.3917577828678,122.238070190751,-107.085978395435));
#25148=CARTESIAN_POINT('Ctrl Pts',(-66.4859783954351,122.238070190751,-106.991757782868));
#25149=CARTESIAN_POINT('Ctrl Pts',(-66.5801990080023,122.238070190751,-106.897537170301));
#25150=CARTESIAN_POINT('Ctrl Pts',(-66.2975371703006,122.238070190751,-107.180199008002));
#25151=CARTESIAN_POINT('Ctrl Pts',(-66.2973702471606,122.238063828476,-107.180030585505));
#25152=CARTESIAN_POINT('Ctrl Pts',(-66.2972001071489,122.238057382362,-107.179858909386));
#25153=CARTESIAN_POINT('Ctrl Pts',(-66.296971463311,122.23804882687,-107.179628057339));
#25154=CARTESIAN_POINT('Ctrl Pts',(-66.2967191259022,122.238039384803,-107.179373282892));
#25155=CARTESIAN_POINT('Ctrl Pts',(-66.2963956021262,122.238027372131,-107.179046504163));
#25156=CARTESIAN_POINT('Ctrl Pts',(-66.295973543409,122.238012105093,-107.178620026165));
#25157=CARTESIAN_POINT('Ctrl Pts',(-66.2955021853265,122.237995054761,-107.1781437326));
#25158=CARTESIAN_POINT('Ctrl Pts',(-66.2949084001559,122.237973979824,-107.17754356376));
#25159=CARTESIAN_POINT('Ctrl Pts',(-66.2942060222409,122.237950147598,-107.176833440411));
#25160=CARTESIAN_POINT('Ctrl Pts',(-66.2933176689234,122.237920005083,-107.175935290825));
#25161=CARTESIAN_POINT('Ctrl Pts',(-66.2922570121511,122.237885609635,-107.1748626695));
#25162=CARTESIAN_POINT('Ctrl Pts',(-66.2911193310074,122.237851483799,-107.173711822738));
#25163=CARTESIAN_POINT('Ctrl Pts',(-66.289971119675,122.2378170421,-107.17255032393));
#25164=CARTESIAN_POINT('Ctrl Pts',(-66.2887498553889,122.237783080562,-107.171314608223));
#25165=CARTESIAN_POINT('Ctrl Pts',(-66.2875548864529,122.237752675088,-107.17010513109));
#25166=CARTESIAN_POINT('Ctrl Pts',(-66.2866600217435,122.237729905638,-107.169199401769));
#25167=CARTESIAN_POINT('Ctrl Pts',(-66.2857804315056,122.237709074602,-107.168308923963));
#25168=CARTESIAN_POINT('Ctrl Pts',(-66.2849305199686,122.237690299368,-107.167448288609));
#25169=CARTESIAN_POINT('Ctrl Pts',(-66.2841588558709,122.237673252684,-107.166666887987));
#25170=CARTESIAN_POINT('Ctrl Pts',(-66.2834120480798,122.237657876347,-107.165910483895));
#25171=CARTESIAN_POINT('Ctrl Pts',(-66.2826693399044,122.237643618104,-107.165158111389));
#25172=CARTESIAN_POINT('Ctrl Pts',(-66.2818923918083,122.237628702536,-107.164371053423));
#25173=CARTESIAN_POINT('Ctrl Pts',(-66.2811127516211,122.237614869895,-107.163581145576));
#25174=CARTESIAN_POINT('Ctrl Pts',(-66.2803056659855,122.237601821719,-107.162763400101));
#25175=CARTESIAN_POINT('Ctrl Pts',(-66.2794046193424,122.237587254472,-107.161850452599));
#25176=CARTESIAN_POINT('Ctrl Pts',(-66.2784699201151,122.237573726381,-107.160903370179));
#25177=CARTESIAN_POINT('Ctrl Pts',(-66.2775198964746,122.237561764432,-107.159940788541));
#25178=CARTESIAN_POINT('Ctrl Pts',(-66.276277873397,122.237546125856,-107.158682347638));
#25179=CARTESIAN_POINT('Ctrl Pts',(-66.2750113535215,122.237533328235,-107.15739913427));
#25180=CARTESIAN_POINT('Ctrl Pts',(-66.2738338670477,122.237524073618,-107.156206223437));
#25181=CARTESIAN_POINT('Ctrl Pts',(-66.27287167512,122.237516511138,-107.155231427378));
#25182=CARTESIAN_POINT('Ctrl Pts',(-66.2719721616253,122.237511277906,-107.154320197339));
#25183=CARTESIAN_POINT('Ctrl Pts',(-66.2711950841845,122.237507801652,-107.153533069771));
#25184=CARTESIAN_POINT('Ctrl Pts',(-66.2705184152976,122.237504774575,-107.152847649364));
#25185=CARTESIAN_POINT('Ctrl Pts',(-66.2699354824588,122.237503040519,-107.152257239457));
#25186=CARTESIAN_POINT('Ctrl Pts',(-66.2694615957603,122.237501974327,-107.15177733498));
#25187=CARTESIAN_POINT('Ctrl Pts',(-66.2690235843036,122.237500988851,-107.151333761317));
#25188=CARTESIAN_POINT('Ctrl Pts',(-66.2686792256979,122.237500559908,-107.150985093111));
#25189=CARTESIAN_POINT('Ctrl Pts',(-66.2684094978787,122.237500316879,-107.150712044098));
#25190=CARTESIAN_POINT('Ctrl Pts',(-66.2681588971757,122.237500091084,-107.150458357716));
#25191=CARTESIAN_POINT('Ctrl Pts',(-66.2679729332289,122.237500027304,-107.150270163797));
#25192=CARTESIAN_POINT('Ctrl Pts',(-66.2678037667766,122.237500006124,-107.150098987781));
#25193=CARTESIAN_POINT('Ctrl Pts',(-66.2677708050049,122.237500001997,-107.150065634449));
#25194=CARTESIAN_POINT('Ctrl Pts',(-66.2677383699138,122.2375,-107.15003281473));
#25195=CARTESIAN_POINT('Ctrl Pts',(-66.2677059397485,122.2375,-107.15));
#25196=CARTESIAN_POINT('Ctrl Pts',(-66.2975371703006,122.238070190751,-107.180199008002));
#25197=CARTESIAN_POINT('Ctrl Pts',(-66.4934491246469,122.245537374399,-107.377870706314));
#25198=CARTESIAN_POINT('Ctrl Pts',(-66.8258653915954,122.385328730462,-107.689134316539));
#25199=CARTESIAN_POINT('Ctrl Pts',(-67.1039244106735,122.739701425857,-107.916794348272));
#25200=CARTESIAN_POINT('Ctrl Pts',(-67.15,122.939812298928,-107.95));
#25201=CARTESIAN_POINT('Ctrl Pts',(-67.15,123.0375,-107.95));
#25202=CARTESIAN_POINT('Ctrl Pts',(-66.3917577828678,122.238070190751,-107.085978395435));
#25203=CARTESIAN_POINT('Ctrl Pts',(-66.5882563185361,122.245537374399,-107.283063512425));
#25204=CARTESIAN_POINT('Ctrl Pts',(-66.9136216999101,122.385328730462,-107.601378008225));
#25205=CARTESIAN_POINT('Ctrl Pts',(-67.1748810565397,122.739701425857,-107.845837702406));
#25206=CARTESIAN_POINT('Ctrl Pts',(-67.2166666666667,122.939812298928,-107.883333333333));
#25207=CARTESIAN_POINT('Ctrl Pts',(-67.2166666666667,123.0375,-107.883333333333));
#25208=CARTESIAN_POINT('Ctrl Pts',(-66.4859783954351,122.238070190751,-106.991757782868));
#25209=CARTESIAN_POINT('Ctrl Pts',(-66.6830635124252,122.245537374399,-107.188256318536));
#25210=CARTESIAN_POINT('Ctrl Pts',(-67.0013780082248,122.385328730462,-107.51362169991));
#25211=CARTESIAN_POINT('Ctrl Pts',(-67.2458377024059,122.739701425857,-107.77488105654));
#25212=CARTESIAN_POINT('Ctrl Pts',(-67.2833333333333,122.939812298928,-107.816666666667));
#25213=CARTESIAN_POINT('Ctrl Pts',(-67.2833333333333,123.0375,-107.816666666667));
#25214=CARTESIAN_POINT('Ctrl Pts',(-66.5801990080023,122.238070190751,-106.897537170301));
#25215=CARTESIAN_POINT('Ctrl Pts',(-66.7778707063143,122.245537374399,-107.093449124647));
#25216=CARTESIAN_POINT('Ctrl Pts',(-67.0891343165395,122.385328730462,-107.425865391595));
#25217=CARTESIAN_POINT('Ctrl Pts',(-67.3167943482721,122.739701425857,-107.703924410673));
#25218=CARTESIAN_POINT('Ctrl Pts',(-67.35,122.939812298928,-107.75));
#25219=CARTESIAN_POINT('Ctrl Pts',(-67.35,123.0375,-107.75));
#25220=CARTESIAN_POINT('',(-67.15,123.0375,-107.95));
#25221=CARTESIAN_POINT('',(-67.35,123.0375,-107.75));
#25222=CARTESIAN_POINT('Ctrl Pts',(-67.15,123.0375,-107.95));
#25223=CARTESIAN_POINT('Ctrl Pts',(-67.15,122.939812298928,-107.95));
#25224=CARTESIAN_POINT('Ctrl Pts',(-67.1039244106735,122.739701425857,-107.916794348272));
#25225=CARTESIAN_POINT('Ctrl Pts',(-66.8258653915954,122.385328730462,-107.689134316539));
#25226=CARTESIAN_POINT('Ctrl Pts',(-66.4934491246469,122.245537374399,-107.377870706314));
#25227=CARTESIAN_POINT('Ctrl Pts',(-66.2975371703006,122.238070190751,-107.180199008002));
#25228=CARTESIAN_POINT('Origin',(-67.25,122.2375,-107.85));
#25229=CARTESIAN_POINT('',(-67.15,126.2,-107.95));
#25230=CARTESIAN_POINT('',(-67.35,126.2,-107.75));
#25231=CARTESIAN_POINT('',(-67.15,122.2375,-107.95));
#25232=CARTESIAN_POINT('Ctrl Pts',(-66.5801990080024,126.999429809249,-106.897537170301));
#25233=CARTESIAN_POINT('Ctrl Pts',(-66.7778707063143,126.991962625601,-107.093449124647));
#25234=CARTESIAN_POINT('Ctrl Pts',(-67.0891344719334,126.852171342114,-107.425865686481));
#25235=CARTESIAN_POINT('Ctrl Pts',(-67.3167946468525,126.497798963876,-107.703924706682));
#25236=CARTESIAN_POINT('Ctrl Pts',(-67.35,126.297687701072,-107.75));
#25237=CARTESIAN_POINT('Ctrl Pts',(-67.35,126.2,-107.75));
#25238=CARTESIAN_POINT('Ctrl Pts',(-66.4859783954351,126.999429809249,-106.991757782868));
#25239=CARTESIAN_POINT('Ctrl Pts',(-66.6830635124252,126.991962625601,-107.188256318536));
#25240=CARTESIAN_POINT('Ctrl Pts',(-67.0013782101158,126.852171342114,-107.513621948298));
#25241=CARTESIAN_POINT('Ctrl Pts',(-67.2458380001291,126.497798963876,-107.774881353406));
#25242=CARTESIAN_POINT('Ctrl Pts',(-67.2833333333333,126.297687701072,-107.816666666667));
#25243=CARTESIAN_POINT('Ctrl Pts',(-67.2833333333333,126.2,-107.816666666667));
#25244=CARTESIAN_POINT('Ctrl Pts',(-66.3917577828678,126.999429809249,-107.085978395435));
#25245=CARTESIAN_POINT('Ctrl Pts',(-66.5882563185361,126.991962625601,-107.283063512425));
#25246=CARTESIAN_POINT('Ctrl Pts',(-66.9136219482982,126.852171342114,-107.601378210116));
#25247=CARTESIAN_POINT('Ctrl Pts',(-67.1748813534057,126.497798963876,-107.845838000129));
#25248=CARTESIAN_POINT('Ctrl Pts',(-67.2166666666667,126.297687701072,-107.883333333333));
#25249=CARTESIAN_POINT('Ctrl Pts',(-67.2166666666667,126.2,-107.883333333333));
#25250=CARTESIAN_POINT('Ctrl Pts',(-66.2975371703006,126.999429809249,-107.180199008002));
#25251=CARTESIAN_POINT('Ctrl Pts',(-66.4934491246469,126.991962625601,-107.377870706314));
#25252=CARTESIAN_POINT('Ctrl Pts',(-66.8258656864805,126.852171342114,-107.689134471933));
#25253=CARTESIAN_POINT('Ctrl Pts',(-67.1039247066823,126.497798963876,-107.916794646852));
#25254=CARTESIAN_POINT('Ctrl Pts',(-67.15,126.297687701072,-107.95));
#25255=CARTESIAN_POINT('Ctrl Pts',(-67.15,126.2,-107.95));
#25256=CARTESIAN_POINT('Ctrl Pts',(-66.2975371703006,126.999429809249,-107.180199008002));
#25257=CARTESIAN_POINT('Ctrl Pts',(-66.4934491246469,126.991962625601,-107.377870706314));
#25258=CARTESIAN_POINT('Ctrl Pts',(-66.8258656864805,126.852171342114,-107.689134471933));
#25259=CARTESIAN_POINT('Ctrl Pts',(-67.1039247066823,126.497798963876,-107.916794646852));
#25260=CARTESIAN_POINT('Ctrl Pts',(-67.15,126.297687701072,-107.95));
#25261=CARTESIAN_POINT('Ctrl Pts',(-67.15,126.2,-107.95));
#25262=CARTESIAN_POINT('Ctrl Pts',(7.79753717030057,122.238070190751,-107.180199008002));
#25263=CARTESIAN_POINT('Ctrl Pts',(7.79586969465498,122.238006634921,-107.178516554556));
#25264=CARTESIAN_POINT('Ctrl Pts',(7.78366424106801,122.237567818931,-107.166171554764));
#25265=CARTESIAN_POINT('Ctrl Pts',(7.77028435014845,122.23750406825,-107.152607599263));
#25266=CARTESIAN_POINT('Ctrl Pts',(7.76812240830435,122.2375,-107.150421407138));
#25267=CARTESIAN_POINT('Ctrl Pts',(7.76770593974856,122.2375,-107.15));
#25268=CARTESIAN_POINT('Ctrl Pts',(7.89175778286783,122.238070190751,-107.085978395435));
#25269=CARTESIAN_POINT('Ctrl Pts',(7.890085314622,122.238006634921,-107.084300934589));
#25270=CARTESIAN_POINT('Ctrl Pts',(7.87782652967437,122.237567818931,-107.072009266158));
#25271=CARTESIAN_POINT('Ctrl Pts',(7.8643945147263,122.23750406825,-107.058497434685));
#25272=CARTESIAN_POINT('Ctrl Pts',(7.86222207458238,122.2375,-107.05632174086));
#25273=CARTESIAN_POINT('Ctrl Pts',(7.86180395983237,122.2375,-107.055901979916));
#25274=CARTESIAN_POINT('Ctrl Pts',(7.98597839543508,122.238070190751,-106.991757782868));
#25275=CARTESIAN_POINT('Ctrl Pts',(7.98430093458903,122.238006634921,-106.990085314622));
#25276=CARTESIAN_POINT('Ctrl Pts',(7.97196847256973,122.237492684192,-106.977826529674));
#25277=CARTESIAN_POINT('Ctrl Pts',(7.95849177929169,122.237549607091,-106.964394514726));
#25278=CARTESIAN_POINT('Ctrl Pts',(7.9563217408604,122.2375,-106.962222074582));
#25279=CARTESIAN_POINT('Ctrl Pts',(7.95590197991618,122.2375,-106.961803959832));
#25280=CARTESIAN_POINT('Ctrl Pts',(8.08019900800234,122.238070190751,-106.897537170301));
#25281=CARTESIAN_POINT('Ctrl Pts',(8.07851655455605,122.238006634921,-106.895869694655));
#25282=CARTESIAN_POINT('Ctrl Pts',(8.06617155476444,122.237567818931,-106.883664241068));
#25283=CARTESIAN_POINT('Ctrl Pts',(8.05260759926268,122.23750406825,-106.870284350148));
#25284=CARTESIAN_POINT('Ctrl Pts',(8.05042140713842,122.2375,-106.868122408304));
#25285=CARTESIAN_POINT('Ctrl Pts',(8.04999999999999,122.2375,-106.867705939749));
#25286=CARTESIAN_POINT('',(7.79753717030057,122.238070190751,-107.180199008002));
#25287=CARTESIAN_POINT('Ctrl Pts',(7.76770593974857,122.2375,-107.15));
#25288=CARTESIAN_POINT('Ctrl Pts',(7.76787269880524,122.2375,-107.150168736525));
#25289=CARTESIAN_POINT('Ctrl Pts',(7.76804267276228,122.237500039141,-107.150340729475));
#25290=CARTESIAN_POINT('Ctrl Pts',(7.76827111985225,122.237500204467,-107.150571968418));
#25291=CARTESIAN_POINT('Ctrl Pts',(7.76852323938491,122.237500386926,-107.150827169104));
#25292=CARTESIAN_POINT('Ctrl Pts',(7.76884650748517,122.23750071898,-107.15115445911));
#25293=CARTESIAN_POINT('Ctrl Pts',(7.76926826289328,122.237501563317,-107.151581551272));
#25294=CARTESIAN_POINT('Ctrl Pts',(7.76973927920157,122.237502506272,-107.152058527665));
#25295=CARTESIAN_POINT('Ctrl Pts',(7.77033266182064,122.237504104656,-107.152659504951));
#25296=CARTESIAN_POINT('Ctrl Pts',(7.77103459621282,122.237507100231,-107.153370507335));
#25297=CARTESIAN_POINT('Ctrl Pts',(7.77192235659105,122.237510888837,-107.154269736312));
#25298=CARTESIAN_POINT('Ctrl Pts',(7.77298234306013,122.237517016609,-107.155343532233));
#25299=CARTESIAN_POINT('Ctrl Pts',(7.7741193736361,122.237526369906,-107.15649547184));
#25300=CARTESIAN_POINT('Ctrl Pts',(7.77526702434705,122.237535810566,-107.157658170837));
#25301=CARTESIAN_POINT('Ctrl Pts',(7.77648776408678,122.237548536479,-107.158895009794));
#25302=CARTESIAN_POINT('Ctrl Pts',(7.77768232341393,122.237563826519,-107.160105362763));
#25303=CARTESIAN_POINT('Ctrl Pts',(7.77857686922413,122.237575276466,-107.161011735642));
#25304=CARTESIAN_POINT('Ctrl Pts',(7.77945620574639,122.237588088159,-107.161902720355));
#25305=CARTESIAN_POINT('Ctrl Pts',(7.78030595164864,122.237601826337,-107.162763689537));
#25306=CARTESIAN_POINT('Ctrl Pts',(7.78107745853227,122.237614299594,-107.163545386335));
#25307=CARTESIAN_POINT('Ctrl Pts',(7.78182418240277,122.237627497267,-107.164301945286));
#25308=CARTESIAN_POINT('Ctrl Pts',(7.78256688209903,122.237641657879,-107.165054319648));
#25309=CARTESIAN_POINT('Ctrl Pts',(7.78334383168152,122.237656471514,-107.165841390048));
#25310=CARTESIAN_POINT('Ctrl Pts',(7.78412355571779,122.23767247258,-107.166631142476));
#25311=CARTESIAN_POINT('Ctrl Pts',(7.78493080553857,122.237690305677,-107.167448577782));
#25312=CARTESIAN_POINT('Ctrl Pts',(7.78583202415144,122.237710214654,-107.168361167533));
#25313=CARTESIAN_POINT('Ctrl Pts',(7.78676699424957,122.237732447119,-107.169307696962));
#25314=CARTESIAN_POINT('Ctrl Pts',(7.78771736014403,122.237756826023,-107.170269575145));
#25315=CARTESIAN_POINT('Ctrl Pts',(7.78895976347825,122.237788696307,-107.171527028373));
#25316=CARTESIAN_POINT('Ctrl Pts',(7.79022678187039,122.237824333785,-107.172808991137));
#25317=CARTESIAN_POINT('Ctrl Pts',(7.79140481193201,122.237860099073,-107.174000600953));
#25318=CARTESIAN_POINT('Ctrl Pts',(7.79236756925898,122.237889328628,-107.174974456476));
#25319=CARTESIAN_POINT('Ctrl Pts',(7.79326766129812,122.237918483816,-107.175884701856));
#25320=CARTESIAN_POINT('Ctrl Pts',(7.79404526837716,122.237944709538,-107.176670911026));
#25321=CARTESIAN_POINT('Ctrl Pts',(7.79472238066739,122.237967545954,-107.177355513708));
#25322=CARTESIAN_POINT('Ctrl Pts',(7.79530572415215,122.237988087761,-107.177945163436));
#25323=CARTESIAN_POINT('Ctrl Pts',(7.79577996678998,122.238005126535,-107.178424413861));
#25324=CARTESIAN_POINT('Ctrl Pts',(7.79621830381088,122.238020875278,-107.178867379523));
#25325=CARTESIAN_POINT('Ctrl Pts',(7.79656294242096,122.238033598544,-107.179215532937));
#25326=CARTESIAN_POINT('Ctrl Pts',(7.79683290736253,122.238043654136,-107.179488151145));
#25327=CARTESIAN_POINT('Ctrl Pts',(7.79708372689204,122.238052996604,-107.179741435775));
#25328=CARTESIAN_POINT('Ctrl Pts',(7.79726987331101,122.238060029675,-107.179929301389));
#25329=CARTESIAN_POINT('Ctrl Pts',(7.79743920767582,122.238066462969,-107.180100163959));
#25330=CARTESIAN_POINT('Ctrl Pts',(7.79747221525505,122.238067716982,-107.180133469425));
#25331=CARTESIAN_POINT('Ctrl Pts',(7.79750469524612,122.238068952964,-107.180166241246));
#25332=CARTESIAN_POINT('Ctrl Pts',(7.79753717030058,122.238070190751,-107.180199008002));
#25333=CARTESIAN_POINT('',(8.08019900800234,122.238070190751,-106.897537170301));
#25334=CARTESIAN_POINT('Ctrl Pts',(8.08019900800234,122.238070190751,-106.897537170301));
#25335=CARTESIAN_POINT('Ctrl Pts',(7.98597839543508,122.238070190751,-106.991757782868));
#25336=CARTESIAN_POINT('Ctrl Pts',(7.89175778286783,122.238070190751,-107.085978395435));
#25337=CARTESIAN_POINT('Ctrl Pts',(7.79753717030057,122.238070190751,-107.180199008002));
#25338=CARTESIAN_POINT('Ctrl Pts',(8.08019900800234,122.238070190751,-106.897537170301));
#25339=CARTESIAN_POINT('Ctrl Pts',(8.08003058550519,122.238063828476,-106.897370247161));
#25340=CARTESIAN_POINT('Ctrl Pts',(8.07985890938578,122.238057382362,-106.897200107149));
#25341=CARTESIAN_POINT('Ctrl Pts',(8.07962805733886,122.23804882687,-106.896971463311));
#25342=CARTESIAN_POINT('Ctrl Pts',(8.07937328289186,122.238039384803,-106.896719125902));
#25343=CARTESIAN_POINT('Ctrl Pts',(8.0790465041628,122.238027372131,-106.896395602126));
#25344=CARTESIAN_POINT('Ctrl Pts',(8.07862002616534,122.238012105093,-106.895973543409));
#25345=CARTESIAN_POINT('Ctrl Pts',(8.07814373260017,122.237995054761,-106.895502185326));
#25346=CARTESIAN_POINT('Ctrl Pts',(8.07754356376052,122.237973979824,-106.894908400156));
#25347=CARTESIAN_POINT('Ctrl Pts',(8.07683344041101,122.237950147598,-106.894206022241));
#25348=CARTESIAN_POINT('Ctrl Pts',(8.07593529082528,122.237920005083,-106.893317668923));
#25349=CARTESIAN_POINT('Ctrl Pts',(8.07486266949997,122.237885609635,-106.892257012151));
#25350=CARTESIAN_POINT('Ctrl Pts',(8.07371182273889,122.237851483799,-106.891119331008));
#25351=CARTESIAN_POINT('Ctrl Pts',(8.07255032393007,122.2378170421,-106.889971119675));
#25352=CARTESIAN_POINT('Ctrl Pts',(8.07131460822295,122.237783080562,-106.888749855389));
#25353=CARTESIAN_POINT('Ctrl Pts',(8.07010513109027,122.237752675088,-106.887554886453));
#25354=CARTESIAN_POINT('Ctrl Pts',(8.06919940176948,122.237729905638,-106.886660021744));
#25355=CARTESIAN_POINT('Ctrl Pts',(8.06830892396311,122.237709074602,-106.885780431506));
#25356=CARTESIAN_POINT('Ctrl Pts',(8.06744828860957,122.237690299368,-106.884930519969));
#25357=CARTESIAN_POINT('Ctrl Pts',(8.06666688798671,122.237673252684,-106.88415885587));
#25358=CARTESIAN_POINT('Ctrl Pts',(8.06591048389357,122.237657876347,-106.883412048079));
#25359=CARTESIAN_POINT('Ctrl Pts',(8.06515811138706,122.237643618104,-106.882669339902));
#25360=CARTESIAN_POINT('Ctrl Pts',(8.06437105342106,122.237628702536,-106.881892391806));
#25361=CARTESIAN_POINT('Ctrl Pts',(8.06358114557415,122.237614869895,-106.881112751619));
#25362=CARTESIAN_POINT('Ctrl Pts',(8.06276340009909,122.237601821719,-106.880305665983));
#25363=CARTESIAN_POINT('Ctrl Pts',(8.06185045259669,122.237587254472,-106.87940461934));
#25364=CARTESIAN_POINT('Ctrl Pts',(8.06090337017639,122.237573726381,-106.878469920113));
#25365=CARTESIAN_POINT('Ctrl Pts',(8.05994078853847,122.237561764432,-106.877519896472));
#25366=CARTESIAN_POINT('Ctrl Pts',(8.05868234763433,122.237546125856,-106.876277873393));
#25367=CARTESIAN_POINT('Ctrl Pts',(8.0573991342653,122.237533328235,-106.875011353517));
#25368=CARTESIAN_POINT('Ctrl Pts',(8.05620622343127,122.237524073618,-106.873833867042));
#25369=CARTESIAN_POINT('Ctrl Pts',(8.05523142737274,122.237516511138,-106.872871675115));
#25370=CARTESIAN_POINT('Ctrl Pts',(8.05432019733458,122.237511277906,-106.871972161621));
#25371=CARTESIAN_POINT('Ctrl Pts',(8.0535330697671,122.237507801652,-106.871195084181));
#25372=CARTESIAN_POINT('Ctrl Pts',(8.05284764936096,122.237504774575,-106.870518415294));
#25373=CARTESIAN_POINT('Ctrl Pts',(8.0522572394541,122.237503040519,-106.869935482456));
#25374=CARTESIAN_POINT('Ctrl Pts',(8.05177733497778,122.237501974327,-106.869461595758));
#25375=CARTESIAN_POINT('Ctrl Pts',(8.0513337613147,122.237500988851,-106.869023584302));
#25376=CARTESIAN_POINT('Ctrl Pts',(8.05098509310967,122.237500559908,-106.868679225696));
#25377=CARTESIAN_POINT('Ctrl Pts',(8.05071204409691,122.237500316879,-106.868409497877));
#25378=CARTESIAN_POINT('Ctrl Pts',(8.0504583577151,122.237500091084,-106.868158897175));
#25379=CARTESIAN_POINT('Ctrl Pts',(8.05027016379602,122.237500027304,-106.867972933228));
#25380=CARTESIAN_POINT('Ctrl Pts',(8.0500989877797,122.237500006124,-106.867803766776));
#25381=CARTESIAN_POINT('Ctrl Pts',(8.05006563444842,122.237500001997,-106.867770805004));
#25382=CARTESIAN_POINT('Ctrl Pts',(8.05003281472958,122.2375,-106.867738369914));
#25383=CARTESIAN_POINT('Ctrl Pts',(8.05,122.2375,-106.867705939749));
#25384=CARTESIAN_POINT('Ctrl Pts',(8.08019900800235,126.999429809249,-106.897537170301));
#25385=CARTESIAN_POINT('Ctrl Pts',(8.07851655455606,126.999493365079,-106.895869694655));
#25386=CARTESIAN_POINT('Ctrl Pts',(8.06617173861538,126.999932177505,-106.883664423923));
#25387=CARTESIAN_POINT('Ctrl Pts',(8.05260764696713,126.999995931145,-106.870284397519));
#25388=CARTESIAN_POINT('Ctrl Pts',(8.05042140713843,127.,-106.868122408304));
#25389=CARTESIAN_POINT('Ctrl Pts',(8.05,127.,-106.867705939749));
#25390=CARTESIAN_POINT('Ctrl Pts',(7.9859783954351,126.999429809249,-106.991757782868));
#25391=CARTESIAN_POINT('Ctrl Pts',(7.98430093458904,126.999493365079,-106.990085314622));
#25392=CARTESIAN_POINT('Ctrl Pts',(7.97200945000902,126.999932177505,-106.977826712529));
#25393=CARTESIAN_POINT('Ctrl Pts',(7.95849748238928,126.999995931145,-106.964394562097));
#25394=CARTESIAN_POINT('Ctrl Pts',(7.95632174086041,127.,-106.962222074582));
#25395=CARTESIAN_POINT('Ctrl Pts',(7.95590197991619,127.,-106.961803959832));
#25396=CARTESIAN_POINT('Ctrl Pts',(7.89175778286785,126.999429809249,-107.085978395435));
#25397=CARTESIAN_POINT('Ctrl Pts',(7.89008531462202,126.999493365079,-107.084300934589));
#25398=CARTESIAN_POINT('Ctrl Pts',(7.8778267125293,127.000007333835,-107.071968657262));
#25399=CARTESIAN_POINT('Ctrl Pts',(7.86439456209684,126.999950397908,-107.058491827139));
#25400=CARTESIAN_POINT('Ctrl Pts',(7.86222207458239,127.,-107.05632174086));
#25401=CARTESIAN_POINT('Ctrl Pts',(7.86180395983238,127.,-107.055901979916));
#25402=CARTESIAN_POINT('Ctrl Pts',(7.7975371703006,126.999429809249,-107.180199008002));
#25403=CARTESIAN_POINT('Ctrl Pts',(7.795869694655,126.999493365079,-107.178516554556));
#25404=CARTESIAN_POINT('Ctrl Pts',(7.78366442392293,126.999932177505,-107.166171738615));
#25405=CARTESIAN_POINT('Ctrl Pts',(7.77028439751899,126.999995931145,-107.152607646967));
#25406=CARTESIAN_POINT('Ctrl Pts',(7.76812240830436,127.,-107.150421407138));
#25407=CARTESIAN_POINT('Ctrl Pts',(7.76770593974857,127.,-107.15));
#25408=CARTESIAN_POINT('',(8.05,127.,-106.867705939749));
#25409=CARTESIAN_POINT('',(8.08019900800235,126.999429809249,-106.897537170301));
#25410=CARTESIAN_POINT('Ctrl Pts',(8.05,127.,-106.867705939749));
#25411=CARTESIAN_POINT('Ctrl Pts',(8.05016873652501,127.,-106.867872698805));
#25412=CARTESIAN_POINT('Ctrl Pts',(8.05034072947524,126.999999960859,-106.868042672762));
#25413=CARTESIAN_POINT('Ctrl Pts',(8.05057196841784,126.999999795533,-106.868271119852));
#25414=CARTESIAN_POINT('Ctrl Pts',(8.05082716910411,126.999999613074,-106.868523239385));
#25415=CARTESIAN_POINT('Ctrl Pts',(8.05115445911008,126.99999928102,-106.868846507485));
#25416=CARTESIAN_POINT('Ctrl Pts',(8.0515815512717,126.999998436683,-106.869268262893));
#25417=CARTESIAN_POINT('Ctrl Pts',(8.05205852766472,126.999997493728,-106.869739279202));
#25418=CARTESIAN_POINT('Ctrl Pts',(8.05265950495146,126.999995895344,-106.870332661821));
#25419=CARTESIAN_POINT('Ctrl Pts',(8.05337050733543,126.999992899769,-106.871034596213));
#25420=CARTESIAN_POINT('Ctrl Pts',(8.05426973631222,126.999989111163,-106.871922356591));
#25421=CARTESIAN_POINT('Ctrl Pts',(8.05534353223281,126.999982983391,-106.87298234306));
#25422=CARTESIAN_POINT('Ctrl Pts',(8.05649547184056,126.999973630094,-106.874119373636));
#25423=CARTESIAN_POINT('Ctrl Pts',(8.05765817083721,126.999964189434,-106.875267024347));
#25424=CARTESIAN_POINT('Ctrl Pts',(8.05889500979385,126.999951463521,-106.876487764087));
#25425=CARTESIAN_POINT('Ctrl Pts',(8.06010536276288,126.999936173481,-106.877682323414));
#25426=CARTESIAN_POINT('Ctrl Pts',(8.06101173564262,126.999924723534,-106.878576869224));
#25427=CARTESIAN_POINT('Ctrl Pts',(8.06190272035554,126.999911911841,-106.879456205747));
#25428=CARTESIAN_POINT('Ctrl Pts',(8.06276368953774,126.999898173663,-106.880305951649));
#25429=CARTESIAN_POINT('Ctrl Pts',(8.0635453863377,126.999885700406,-106.881077458535));
#25430=CARTESIAN_POINT('Ctrl Pts',(8.06430194529093,126.999872502733,-106.881824182407));
#25431=CARTESIAN_POINT('Ctrl Pts',(8.0650543196552,126.99985834212,-106.882566882106));
#25432=CARTESIAN_POINT('Ctrl Pts',(8.06584139005466,126.999843528486,-106.883343831688));
#25433=CARTESIAN_POINT('Ctrl Pts',(8.06663114248294,126.99982752742,-106.884123555725));
#25434=CARTESIAN_POINT('Ctrl Pts',(8.06744857778991,126.999809694323,-106.884930805546));
#25435=CARTESIAN_POINT('Ctrl Pts',(8.06836116754174,126.999789785345,-106.885832024159));
#25436=CARTESIAN_POINT('Ctrl Pts',(8.0693076969708,126.999767552881,-106.886766994258));
#25437=CARTESIAN_POINT('Ctrl Pts',(8.07026957515425,126.999743173977,-106.887717360153));
#25438=CARTESIAN_POINT('Ctrl Pts',(8.07152702838454,126.999711303692,-106.88895976349));
#25439=CARTESIAN_POINT('Ctrl Pts',(8.07280899115145,126.999675666215,-106.890226781884));
#25440=CARTESIAN_POINT('Ctrl Pts',(8.07400060096861,126.999639900926,-106.891404811947));
#25441=CARTESIAN_POINT('Ctrl Pts',(8.07497445648938,126.999610671372,-106.892367569273));
#25442=CARTESIAN_POINT('Ctrl Pts',(8.07588470186807,126.999581516183,-106.89326766131));
#25443=CARTESIAN_POINT('Ctrl Pts',(8.0766709110366,126.999555290461,-106.894045268387));
#25444=CARTESIAN_POINT('Ctrl Pts',(8.07735551371743,126.999532454045,-106.894722380676));
#25445=CARTESIAN_POINT('Ctrl Pts',(8.07794516344381,126.999511912239,-106.89530572416));
#25446=CARTESIAN_POINT('Ctrl Pts',(8.07842441386779,126.999494873465,-106.895779966796));
#25447=CARTESIAN_POINT('Ctrl Pts',(8.07886737952789,126.999479124722,-106.896218303816));
#25448=CARTESIAN_POINT('Ctrl Pts',(8.07921553294167,126.999466401456,-106.896562942425));
#25449=CARTESIAN_POINT('Ctrl Pts',(8.07948815114815,126.999456345864,-106.896832907366));
#25450=CARTESIAN_POINT('Ctrl Pts',(8.07974143577804,126.999447003396,-106.897083726895));
#25451=CARTESIAN_POINT('Ctrl Pts',(8.07992930139156,126.999439970325,-106.897269873313));
#25452=CARTESIAN_POINT('Ctrl Pts',(8.08010016396172,126.999433537031,-106.897439207678));
#25453=CARTESIAN_POINT('Ctrl Pts',(8.08013346942631,126.999432283018,-106.897472215257));
#25454=CARTESIAN_POINT('Ctrl Pts',(8.08016624124731,126.999431047035,-106.897504695247));
#25455=CARTESIAN_POINT('Ctrl Pts',(8.08019900800235,126.999429809249,-106.897537170301));
#25456=CARTESIAN_POINT('',(7.7975371703006,126.999429809249,-107.180199008002));
#25457=CARTESIAN_POINT('Ctrl Pts',(7.7975371703006,126.999429809249,-107.180199008002));
#25458=CARTESIAN_POINT('Ctrl Pts',(7.89175778286785,126.999429809249,-107.085978395435));
#25459=CARTESIAN_POINT('Ctrl Pts',(7.9859783954351,126.999429809249,-106.991757782868));
#25460=CARTESIAN_POINT('Ctrl Pts',(8.08019900800235,126.999429809249,-106.897537170301));
#25461=CARTESIAN_POINT('',(7.76770593974857,127.,-107.15));
#25462=CARTESIAN_POINT('Ctrl Pts',(7.7975371703006,126.999429809249,-107.180199008002));
#25463=CARTESIAN_POINT('Ctrl Pts',(7.7973702471606,126.999436171524,-107.180030585505));
#25464=CARTESIAN_POINT('Ctrl Pts',(7.79720010714892,126.999442617638,-107.179858909386));
#25465=CARTESIAN_POINT('Ctrl Pts',(7.79697146331107,126.99945117313,-107.179628057339));
#25466=CARTESIAN_POINT('Ctrl Pts',(7.79671912590221,126.999460615197,-107.179373282892));
#25467=CARTESIAN_POINT('Ctrl Pts',(7.79639560212622,126.999472627869,-107.179046504163));
#25468=CARTESIAN_POINT('Ctrl Pts',(7.79597354340904,126.999487894907,-107.178620026165));
#25469=CARTESIAN_POINT('Ctrl Pts',(7.79550218532651,126.999504945239,-107.1781437326));
#25470=CARTESIAN_POINT('Ctrl Pts',(7.79490840015591,126.999526020176,-107.177543563761));
#25471=CARTESIAN_POINT('Ctrl Pts',(7.79420602224097,126.999549852402,-107.176833440411));
#25472=CARTESIAN_POINT('Ctrl Pts',(7.79331766892345,126.999579994917,-107.175935290825));
#25473=CARTESIAN_POINT('Ctrl Pts',(7.79225701215115,126.999614390365,-107.1748626695));
#25474=CARTESIAN_POINT('Ctrl Pts',(7.7911193310075,126.999648516201,-107.173711822739));
#25475=CARTESIAN_POINT('Ctrl Pts',(7.78997111967503,126.9996829579,-107.17255032393));
#25476=CARTESIAN_POINT('Ctrl Pts',(7.78874985538896,126.999716919438,-107.171314608223));
#25477=CARTESIAN_POINT('Ctrl Pts',(7.78755488645297,126.999747324912,-107.17010513109));
#25478=CARTESIAN_POINT('Ctrl Pts',(7.78666002174368,126.999770094362,-107.169199401769));
#25479=CARTESIAN_POINT('Ctrl Pts',(7.78578043150578,126.999790925398,-107.168308923963));
#25480=CARTESIAN_POINT('Ctrl Pts',(7.78493051996893,126.999809700632,-107.167448288609));
#25481=CARTESIAN_POINT('Ctrl Pts',(7.78415885587109,126.999826747316,-107.166666887987));
#25482=CARTESIAN_POINT('Ctrl Pts',(7.78341204807995,126.999842123653,-107.165910483895));
#25483=CARTESIAN_POINT('Ctrl Pts',(7.78266933990444,126.999856381896,-107.165158111389));
#25484=CARTESIAN_POINT('Ctrl Pts',(7.78189239180835,126.999871297464,-107.164371053423));
#25485=CARTESIAN_POINT('Ctrl Pts',(7.78111275162114,126.999885130105,-107.163581145576));
#25486=CARTESIAN_POINT('Ctrl Pts',(7.78030566598552,126.999898178281,-107.162763400101));
#25487=CARTESIAN_POINT('Ctrl Pts',(7.77940461934248,126.999912745528,-107.161850452599));
#25488=CARTESIAN_POINT('Ctrl Pts',(7.77846992011515,126.999926273619,-107.160903370179));
#25489=CARTESIAN_POINT('Ctrl Pts',(7.77751989647463,126.999938235568,-107.159940788541));
#25490=CARTESIAN_POINT('Ctrl Pts',(7.77627787339686,126.999953874144,-107.158682347638));
#25491=CARTESIAN_POINT('Ctrl Pts',(7.77501135352116,126.999966671765,-107.15739913427));
#25492=CARTESIAN_POINT('Ctrl Pts',(7.77383386704725,126.999975926382,-107.156206223436));
#25493=CARTESIAN_POINT('Ctrl Pts',(7.77287167511962,126.999983488862,-107.155231427377));
#25494=CARTESIAN_POINT('Ctrl Pts',(7.771972161625,126.999988722094,-107.154320197339));
#25495=CARTESIAN_POINT('Ctrl Pts',(7.77119508418426,126.999992198348,-107.153533069771));
#25496=CARTESIAN_POINT('Ctrl Pts',(7.77051841529733,126.999995225425,-107.152847649364));
#25497=CARTESIAN_POINT('Ctrl Pts',(7.76993548245859,126.999996959481,-107.152257239457));
#25498=CARTESIAN_POINT('Ctrl Pts',(7.76946159576003,126.999998025673,-107.15177733498));
#25499=CARTESIAN_POINT('Ctrl Pts',(7.7690235843034,126.999999011149,-107.151333761317));
#25500=CARTESIAN_POINT('Ctrl Pts',(7.76867922569782,126.999999440092,-107.150985093111));
#25501=CARTESIAN_POINT('Ctrl Pts',(7.76840949787861,126.999999683121,-107.150712044098));
#25502=CARTESIAN_POINT('Ctrl Pts',(7.76815889717565,126.999999908916,-107.150458357716));
#25503=CARTESIAN_POINT('Ctrl Pts',(7.76797293322885,126.999999972695,-107.150270163797));
#25504=CARTESIAN_POINT('Ctrl Pts',(7.76780376677657,126.999999993876,-107.150098987781));
#25505=CARTESIAN_POINT('Ctrl Pts',(7.76777080500488,126.999999998003,-107.150065634449));
#25506=CARTESIAN_POINT('Ctrl Pts',(7.76773836991385,127.,-107.15003281473));
#25507=CARTESIAN_POINT('Ctrl Pts',(7.76770593974857,127.,-107.15));
#25508=CARTESIAN_POINT('',(7.90885296987428,127.,-107.008852969874));
#25509=CARTESIAN_POINT('Ctrl Pts',(7.7975371703006,126.999429809249,-107.180199008002));
#25510=CARTESIAN_POINT('Ctrl Pts',(7.99344912464694,126.991962625601,-107.377870706314));
#25511=CARTESIAN_POINT('Ctrl Pts',(8.32585953691074,126.852169925683,-107.68913127501));
#25512=CARTESIAN_POINT('Ctrl Pts',(8.60391850229334,126.49779073068,-107.916788359609));
#25513=CARTESIAN_POINT('Ctrl Pts',(8.65,126.297687701072,-107.95));
#25514=CARTESIAN_POINT('Ctrl Pts',(8.64999999999999,126.2,-107.95));
#25515=CARTESIAN_POINT('Ctrl Pts',(7.89175778286785,126.999429809249,-107.085978395435));
#25516=CARTESIAN_POINT('Ctrl Pts',(8.08825631853607,126.991962625601,-107.283063512425));
#25517=CARTESIAN_POINT('Ctrl Pts',(8.413616782944,126.852169925683,-107.601374028977));
#25518=CARTESIAN_POINT('Ctrl Pts',(8.6748751213987,126.49779073068,-107.845831740504));
#25519=CARTESIAN_POINT('Ctrl Pts',(8.71666666666666,126.297687701072,-107.883333333333));
#25520=CARTESIAN_POINT('Ctrl Pts',(8.71666666666666,126.2,-107.883333333333));
#25521=CARTESIAN_POINT('Ctrl Pts',(7.9859783954351,126.999429809249,-106.991757782868));
#25522=CARTESIAN_POINT('Ctrl Pts',(8.18306351242521,126.991962625601,-107.188256318536));
#25523=CARTESIAN_POINT('Ctrl Pts',(8.50137402897724,126.852169925683,-107.513616782944));
#25524=CARTESIAN_POINT('Ctrl Pts',(8.74583174050407,126.49779073068,-107.774875121399));
#25525=CARTESIAN_POINT('Ctrl Pts',(8.78333333333333,126.297687701072,-107.816666666667));
#25526=CARTESIAN_POINT('Ctrl Pts',(8.78333333333333,126.2,-107.816666666667));
#25527=CARTESIAN_POINT('Ctrl Pts',(8.08019900800235,126.999429809249,-106.897537170301));
#25528=CARTESIAN_POINT('Ctrl Pts',(8.27787070631435,126.991962625601,-107.093449124647));
#25529=CARTESIAN_POINT('Ctrl Pts',(8.58913127501049,126.852169925683,-107.425859536911));
#25530=CARTESIAN_POINT('Ctrl Pts',(8.81678835960943,126.49779073068,-107.703918502293));
#25531=CARTESIAN_POINT('Ctrl Pts',(8.85,126.297687701072,-107.75));
#25532=CARTESIAN_POINT('Ctrl Pts',(8.85,126.2,-107.75));
#25533=CARTESIAN_POINT('',(8.85,126.2,-107.75));
#25534=CARTESIAN_POINT('Ctrl Pts',(8.08019900800235,126.999429809249,-106.897537170301));
#25535=CARTESIAN_POINT('Ctrl Pts',(8.27787070631435,126.991962625601,-107.093449124647));
#25536=CARTESIAN_POINT('Ctrl Pts',(8.58913127501049,126.852169925683,-107.425859536911));
#25537=CARTESIAN_POINT('Ctrl Pts',(8.81678835960943,126.49779073068,-107.703918502293));
#25538=CARTESIAN_POINT('Ctrl Pts',(8.85,126.297687701072,-107.75));
#25539=CARTESIAN_POINT('Ctrl Pts',(8.85,126.2,-107.75));
#25540=CARTESIAN_POINT('',(8.64999999999999,126.2,-107.95));
#25541=CARTESIAN_POINT('',(8.85,126.2,-107.75));
#25542=CARTESIAN_POINT('Ctrl Pts',(8.64999999999999,126.2,-107.95));
#25543=CARTESIAN_POINT('Ctrl Pts',(8.65,126.297687701072,-107.95));
#25544=CARTESIAN_POINT('Ctrl Pts',(8.60391850229334,126.49779073068,-107.916788359609));
#25545=CARTESIAN_POINT('Ctrl Pts',(8.32585953691074,126.852169925683,-107.68913127501));
#25546=CARTESIAN_POINT('Ctrl Pts',(7.99344912464694,126.991962625601,-107.377870706314));
#25547=CARTESIAN_POINT('Ctrl Pts',(7.7975371703006,126.999429809249,-107.180199008002));
#25548=CARTESIAN_POINT('Origin',(8.74999999999999,122.2375,-107.85));
#25549=CARTESIAN_POINT('',(8.84999999999999,123.0375,-107.75));
#25550=CARTESIAN_POINT('',(8.84999999999999,122.2375,-107.75));
#25551=CARTESIAN_POINT('',(8.64999999999999,123.0375,-107.95));
#25552=CARTESIAN_POINT('',(8.84999999999999,123.0375,-107.75));
#25553=CARTESIAN_POINT('',(8.64999999999999,122.2375,-107.95));
#25554=CARTESIAN_POINT('Ctrl Pts',(8.08019900800234,122.238070190751,-106.897537170301));
#25555=CARTESIAN_POINT('Ctrl Pts',(8.27787070631434,122.245537374399,-107.093449124647));
#25556=CARTESIAN_POINT('Ctrl Pts',(8.5891310580126,122.38533016425,-107.425859112781));
#25557=CARTESIAN_POINT('Ctrl Pts',(8.81678792114121,122.739709845598,-107.703918071875));
#25558=CARTESIAN_POINT('Ctrl Pts',(8.85,122.939812298928,-107.75));
#25559=CARTESIAN_POINT('Ctrl Pts',(8.85,123.0375,-107.75));
#25560=CARTESIAN_POINT('Ctrl Pts',(7.98597839543508,122.238070190751,-106.991757782868));
#25561=CARTESIAN_POINT('Ctrl Pts',(8.18306351242519,122.245537374399,-107.188256318536));
#25562=CARTESIAN_POINT('Ctrl Pts',(8.50137374293551,122.38533016425,-107.513616427858));
#25563=CARTESIAN_POINT('Ctrl Pts',(8.74583130471913,122.739709845598,-107.774874688297));
#25564=CARTESIAN_POINT('Ctrl Pts',(8.78333333333333,122.939812298928,-107.816666666667));
#25565=CARTESIAN_POINT('Ctrl Pts',(8.78333333333333,123.0375,-107.816666666667));
#25566=CARTESIAN_POINT('Ctrl Pts',(7.89175778286783,122.238070190751,-107.085978395435));
#25567=CARTESIAN_POINT('Ctrl Pts',(8.08825631853605,122.245537374399,-107.283063512425));
#25568=CARTESIAN_POINT('Ctrl Pts',(8.41361642785841,122.38533016425,-107.601373742935));
#25569=CARTESIAN_POINT('Ctrl Pts',(8.67487468829706,122.739709845598,-107.845831304719));
#25570=CARTESIAN_POINT('Ctrl Pts',(8.71666666666666,122.939812298928,-107.883333333333));
#25571=CARTESIAN_POINT('Ctrl Pts',(8.71666666666666,123.0375,-107.883333333333));
#25572=CARTESIAN_POINT('Ctrl Pts',(7.79753717030057,122.238070190751,-107.180199008002));
#25573=CARTESIAN_POINT('Ctrl Pts',(7.99344912464692,122.245537374399,-107.377870706314));
#25574=CARTESIAN_POINT('Ctrl Pts',(8.32585911278131,122.38533016425,-107.689131058013));
#25575=CARTESIAN_POINT('Ctrl Pts',(8.60391807187497,122.739709845598,-107.916787921141));
#25576=CARTESIAN_POINT('Ctrl Pts',(8.65,122.939812298928,-107.95));
#25577=CARTESIAN_POINT('Ctrl Pts',(8.65,123.0375,-107.95));
#25578=CARTESIAN_POINT('Ctrl Pts',(7.79753717030057,122.238070190751,-107.180199008002));
#25579=CARTESIAN_POINT('Ctrl Pts',(7.99344912464692,122.245537374399,-107.377870706314));
#25580=CARTESIAN_POINT('Ctrl Pts',(8.32585911278131,122.38533016425,-107.689131058013));
#25581=CARTESIAN_POINT('Ctrl Pts',(8.60391807187497,122.739709845598,-107.916787921141));
#25582=CARTESIAN_POINT('Ctrl Pts',(8.65,122.939812298928,-107.95));
#25583=CARTESIAN_POINT('Ctrl Pts',(8.65,123.0375,-107.95));
#25584=CARTESIAN_POINT('Ctrl Pts',(8.85,123.0375,-107.75));
#25585=CARTESIAN_POINT('Ctrl Pts',(8.85,122.939812298928,-107.75));
#25586=CARTESIAN_POINT('Ctrl Pts',(8.81678792114121,122.739709845598,-107.703918071875));
#25587=CARTESIAN_POINT('Ctrl Pts',(8.5891310580126,122.38533016425,-107.425859112781));
#25588=CARTESIAN_POINT('Ctrl Pts',(8.27787070631434,122.245537374399,-107.093449124647));
#25589=CARTESIAN_POINT('Ctrl Pts',(8.08019900800234,122.238070190751,-106.897537170301));
#25590=CARTESIAN_POINT('Origin',(8.05,123.0375,6.35000000000001));
#25591=CARTESIAN_POINT('',(8.84999999999999,123.0375,44.25));
#25592=CARTESIAN_POINT('',(8.84999999999999,123.0375,6.35000000000001));
#25593=CARTESIAN_POINT('',(8.08019900800235,122.238070190751,43.3975371703006));
#25594=CARTESIAN_POINT('Ctrl Pts',(8.08019900800235,122.238070190751,43.3975371703006));
#25595=CARTESIAN_POINT('Ctrl Pts',(8.27787070631434,122.245537374399,43.5934491246469));
#25596=CARTESIAN_POINT('Ctrl Pts',(8.5891258667193,122.385332034808,43.9258486625008));
#25597=CARTESIAN_POINT('Ctrl Pts',(8.81677690192765,122.739724420659,44.2039073549789));
#25598=CARTESIAN_POINT('Ctrl Pts',(8.85,122.939812298928,44.25));
#25599=CARTESIAN_POINT('Ctrl Pts',(8.85,123.0375,44.25));
#25600=CARTESIAN_POINT('Ctrl Pts',(8.05,122.2375,43.3677059397486));
#25601=CARTESIAN_POINT('Ctrl Pts',(8.050168736525,122.2375,43.3678726988052));
#25602=CARTESIAN_POINT('Ctrl Pts',(8.05034072947523,122.237500039141,43.3680426727623));
#25603=CARTESIAN_POINT('Ctrl Pts',(8.05057196841782,122.237500204467,43.3682711198522));
#25604=CARTESIAN_POINT('Ctrl Pts',(8.0508271691041,122.237500386926,43.3685232393849));
#25605=CARTESIAN_POINT('Ctrl Pts',(8.05115445911008,122.23750071898,43.3688465074852));
#25606=CARTESIAN_POINT('Ctrl Pts',(8.05158155127172,122.237501563317,43.3692682628933));
#25607=CARTESIAN_POINT('Ctrl Pts',(8.05205852766469,122.237502506272,43.3697392792016));
#25608=CARTESIAN_POINT('Ctrl Pts',(8.05265950495136,122.237504104656,43.3703326618206));
#25609=CARTESIAN_POINT('Ctrl Pts',(8.05337050733524,122.237507100231,43.3710345962128));
#25610=CARTESIAN_POINT('Ctrl Pts',(8.05426973631202,122.237510888837,43.371922356591));
#25611=CARTESIAN_POINT('Ctrl Pts',(8.05534353223261,122.237517016609,43.3729823430601));
#25612=CARTESIAN_POINT('Ctrl Pts',(8.05649547184038,122.237526369906,43.3741193736361));
#25613=CARTESIAN_POINT('Ctrl Pts',(8.05765817083703,122.237535810566,43.375267024347));
#25614=CARTESIAN_POINT('Ctrl Pts',(8.05889500979368,122.237548536479,43.3764877640867));
#25615=CARTESIAN_POINT('Ctrl Pts',(8.06010536276272,122.237563826519,43.3776823234139));
#25616=CARTESIAN_POINT('Ctrl Pts',(8.06101173564243,122.237575276466,43.3785768692241));
#25617=CARTESIAN_POINT('Ctrl Pts',(8.06190272035532,122.237588088159,43.3794562057464));
#25618=CARTESIAN_POINT('Ctrl Pts',(8.0627636895375,122.237601826337,43.3803059516487));
#25619=CARTESIAN_POINT('Ctrl Pts',(8.06354538633161,122.237614299594,43.3810774585288));
#25620=CARTESIAN_POINT('Ctrl Pts',(8.06430194527942,122.237627497267,43.3818241823961));
#25621=CARTESIAN_POINT('Ctrl Pts',(8.06505431963808,122.237641657879,43.3825668820889));
#25622=CARTESIAN_POINT('Ctrl Pts',(8.06584139003716,122.237656471514,43.3833438316712));
#25623=CARTESIAN_POINT('Ctrl Pts',(8.06663114246472,122.23767247258,43.3841235557071));
#25624=CARTESIAN_POINT('Ctrl Pts',(8.06744857777091,122.237690305677,43.3849308055274));
#25625=CARTESIAN_POINT('Ctrl Pts',(8.06836116752135,122.237710214654,43.3858320241394));
#25626=CARTESIAN_POINT('Ctrl Pts',(8.06930769694889,122.237732447118,43.3867669942366));
#25627=CARTESIAN_POINT('Ctrl Pts',(8.07026957513112,122.237756826022,43.3877173601304));
#25628=CARTESIAN_POINT('Ctrl Pts',(8.07152702835507,122.237788696307,43.3889597634607));
#25629=CARTESIAN_POINT('Ctrl Pts',(8.07280899111595,122.237824333784,43.3902267818492));
#25630=CARTESIAN_POINT('Ctrl Pts',(8.07400060092939,122.237860099073,43.3914048119085));
#25631=CARTESIAN_POINT('Ctrl Pts',(8.07497445645421,122.237889328627,43.3923675692379));
#25632=CARTESIAN_POINT('Ctrl Pts',(8.07588470183759,122.237918483816,43.3932676612799));
#25633=CARTESIAN_POINT('Ctrl Pts',(8.07667091101072,122.237944709538,43.3940452683617));
#25634=CARTESIAN_POINT('Ctrl Pts',(8.0773555136947,122.237967545954,43.3947223806538));
#25635=CARTESIAN_POINT('Ctrl Pts',(8.0779451634244,122.237988087761,43.3953057241405));
#25636=CARTESIAN_POINT('Ctrl Pts',(8.0784244138514,122.238005126535,43.3957799667801));
#25637=CARTESIAN_POINT('Ctrl Pts',(8.07886737951421,122.238020875278,43.3962183038026));
#25638=CARTESIAN_POINT('Ctrl Pts',(8.0792155329305,122.238033598544,43.3965629424142));
#25639=CARTESIAN_POINT('Ctrl Pts',(8.07948815113889,122.238043654136,43.3968329073569));
#25640=CARTESIAN_POINT('Ctrl Pts',(8.07974143577039,122.238052996604,43.3970837268874));
#25641=CARTESIAN_POINT('Ctrl Pts',(8.0799293013851,122.238060029674,43.3972698733071));
#25642=CARTESIAN_POINT('Ctrl Pts',(8.08010016395565,122.238066462969,43.3974392076721));
#25643=CARTESIAN_POINT('Ctrl Pts',(8.08013346942233,122.238067716982,43.3974722152526));
#25644=CARTESIAN_POINT('Ctrl Pts',(8.08016624124532,122.238068952964,43.3975046952449));
#25645=CARTESIAN_POINT('Ctrl Pts',(8.08019900800235,122.238070190751,43.3975371703006));
#25646=CARTESIAN_POINT('Origin',(8.84999999999999,122.2375,44.45));
#25647=CARTESIAN_POINT('',(8.85,126.2,44.25));
#25648=CARTESIAN_POINT('',(8.84999999999999,126.2,6.35000000000001));
#25649=CARTESIAN_POINT('',(8.84999999999999,122.2375,44.25));
#25650=CARTESIAN_POINT('Origin',(8.05,126.2,6.35000000000001));
#25651=CARTESIAN_POINT('',(8.05,127.,43.3677059397486));
#25652=CARTESIAN_POINT('',(8.05,127.,6.35000000000001));
#25653=CARTESIAN_POINT('',(8.08019900800234,126.999429809249,43.3975371703006));
#25654=CARTESIAN_POINT('Ctrl Pts',(8.08019900800234,126.999429809249,43.3975371703006));
#25655=CARTESIAN_POINT('Ctrl Pts',(8.0800305855052,126.999436171524,43.3973702471606));
#25656=CARTESIAN_POINT('Ctrl Pts',(8.0798589093858,126.999442617638,43.3972001071489));
#25657=CARTESIAN_POINT('Ctrl Pts',(8.07962805733889,126.99945117313,43.3969714633111));
#25658=CARTESIAN_POINT('Ctrl Pts',(8.0793732828919,126.999460615197,43.3967191259022));
#25659=CARTESIAN_POINT('Ctrl Pts',(8.07904650416285,126.999472627869,43.3963956021262));
#25660=CARTESIAN_POINT('Ctrl Pts',(8.0786200261654,126.999487894907,43.395973543409));
#25661=CARTESIAN_POINT('Ctrl Pts',(8.07814373260023,126.999504945239,43.3955021853265));
#25662=CARTESIAN_POINT('Ctrl Pts',(8.07754356376057,126.999526020176,43.3949084001559));
#25663=CARTESIAN_POINT('Ctrl Pts',(8.07683344041104,126.999549852402,43.3942060222409));
#25664=CARTESIAN_POINT('Ctrl Pts',(8.07593529082521,126.999579994917,43.3933176689234));
#25665=CARTESIAN_POINT('Ctrl Pts',(8.07486266949977,126.999614390365,43.3922570121511));
#25666=CARTESIAN_POINT('Ctrl Pts',(8.07371182273854,126.999648516201,43.3911193310075));
#25667=CARTESIAN_POINT('Ctrl Pts',(8.07255032392972,126.9996829579,43.389971119675));
#25668=CARTESIAN_POINT('Ctrl Pts',(8.07131460822261,126.999716919438,43.3887498553889));
#25669=CARTESIAN_POINT('Ctrl Pts',(8.07010513108995,126.999747324912,43.3875548864529));
#25670=CARTESIAN_POINT('Ctrl Pts',(8.06919940176919,126.999770094362,43.3866600217436));
#25671=CARTESIAN_POINT('Ctrl Pts',(8.06830892396286,126.999790925398,43.3857804315057));
#25672=CARTESIAN_POINT('Ctrl Pts',(8.06744828860937,126.999809700632,43.3849305199689));
#25673=CARTESIAN_POINT('Ctrl Pts',(8.06666688798462,126.999826747316,43.3841588558684));
#25674=CARTESIAN_POINT('Ctrl Pts',(8.06591048388973,126.999842123653,43.3834120480748));
#25675=CARTESIAN_POINT('Ctrl Pts',(8.06515811138141,126.999856381896,43.3826693398968));
#25676=CARTESIAN_POINT('Ctrl Pts',(8.06437105341527,126.999871297464,43.3818923918005));
#25677=CARTESIAN_POINT('Ctrl Pts',(8.0635811455681,126.999885130105,43.381112751613));
#25678=CARTESIAN_POINT('Ctrl Pts',(8.06276340009277,126.999898178282,43.380305665977));
#25679=CARTESIAN_POINT('Ctrl Pts',(8.06185045258994,126.999912745528,43.3794046193334));
#25680=CARTESIAN_POINT('Ctrl Pts',(8.06090337016919,126.999926273619,43.3784699201053));
#25681=CARTESIAN_POINT('Ctrl Pts',(8.0599407885309,126.999938235568,43.3775198964643));
#25682=CARTESIAN_POINT('Ctrl Pts',(8.05868234762488,126.999953874144,43.3762778733838));
#25683=CARTESIAN_POINT('Ctrl Pts',(8.05739913425408,126.999966671765,43.3750113535055));
#25684=CARTESIAN_POINT('Ctrl Pts',(8.05620622341898,126.999975926382,43.37383386703));
#25685=CARTESIAN_POINT('Ctrl Pts',(8.05523142736173,126.999983488862,43.3728716751042));
#25686=CARTESIAN_POINT('Ctrl Pts',(8.05432019732505,126.999988722094,43.3719721616116));
#25687=CARTESIAN_POINT('Ctrl Pts',(8.05353306975903,126.999992198348,43.3711950841729));
#25688=CARTESIAN_POINT('Ctrl Pts',(8.05284764935386,126.999995225425,43.3705184152873));
#25689=CARTESIAN_POINT('Ctrl Pts',(8.05225723944801,126.999996959481,43.36993548245));
#25690=CARTESIAN_POINT('Ctrl Pts',(8.05177733497262,126.999998025673,43.3694615957528));
#25691=CARTESIAN_POINT('Ctrl Pts',(8.05133376131042,126.999999011149,43.3690235842973));
#25692=CARTESIAN_POINT('Ctrl Pts',(8.0509850931062,126.999999440092,43.3686792256928));
#25693=CARTESIAN_POINT('Ctrl Pts',(8.05071204409405,126.999999683121,43.3684094978744));
#25694=CARTESIAN_POINT('Ctrl Pts',(8.0504583577127,126.999999908916,43.3681588971722));
#25695=CARTESIAN_POINT('Ctrl Pts',(8.05027016379399,126.999999972695,43.3679729332259));
#25696=CARTESIAN_POINT('Ctrl Pts',(8.05009898777776,126.999999993876,43.3678037667738));
#25697=CARTESIAN_POINT('Ctrl Pts',(8.05006563444715,126.999999998003,43.3677708050031));
#25698=CARTESIAN_POINT('Ctrl Pts',(8.05003281472894,127.,43.3677383699129));
#25699=CARTESIAN_POINT('Ctrl Pts',(8.05,127.,43.3677059397486));
#25700=CARTESIAN_POINT('Ctrl Pts',(8.85,126.2,44.25));
#25701=CARTESIAN_POINT('Ctrl Pts',(8.85,126.297687701072,44.25));
#25702=CARTESIAN_POINT('Ctrl Pts',(8.81677764270249,126.497776564831,44.2039080692991));
#25703=CARTESIAN_POINT('Ctrl Pts',(8.58912619963984,126.852168067061,43.9258493522423));
#25704=CARTESIAN_POINT('Ctrl Pts',(8.27787070631434,126.991962625601,43.5934491246469));
#25705=CARTESIAN_POINT('Ctrl Pts',(8.08019900800234,126.999429809249,43.3975371703006));
#25706=CARTESIAN_POINT('Origin',(-29.25,127.,-31.75));
#25707=CARTESIAN_POINT('',(7.76770593974856,127.,43.65));
#25708=CARTESIAN_POINT('',(-48.3,127.,43.65));
#25709=CARTESIAN_POINT('',(7.90885296987428,127.,43.5088529698743));
#25710=CARTESIAN_POINT('',(-10.2,127.,-107.15));
#25711=CARTESIAN_POINT('Ctrl Pts',(8.08019900800235,122.238070190751,43.3975371703006));
#25712=CARTESIAN_POINT('Ctrl Pts',(8.07851655455606,122.238006634921,43.395869694655));
#25713=CARTESIAN_POINT('Ctrl Pts',(8.06616819355892,122.2375677537,43.3836608980584));
#25714=CARTESIAN_POINT('Ctrl Pts',(8.05260673028965,122.237504057297,43.3702834872759));
#25715=CARTESIAN_POINT('Ctrl Pts',(8.05042140713843,122.2375,43.3681224083044));
#25716=CARTESIAN_POINT('Ctrl Pts',(8.05,122.2375,43.3677059397486));
#25717=CARTESIAN_POINT('Ctrl Pts',(7.98597839543509,122.238070190751,43.4917577828678));
#25718=CARTESIAN_POINT('Ctrl Pts',(7.98430093458904,122.238006634921,43.490085314622));
#25719=CARTESIAN_POINT('Ctrl Pts',(7.97200590495255,122.2375677537,43.4778231866648));
#25720=CARTESIAN_POINT('Ctrl Pts',(7.95849656571179,122.237504057297,43.4643936518537));
#25721=CARTESIAN_POINT('Ctrl Pts',(7.9563217408604,122.2375,43.4622220745824));
#25722=CARTESIAN_POINT('Ctrl Pts',(7.95590197991618,122.2375,43.4618039598324));
#25723=CARTESIAN_POINT('Ctrl Pts',(7.89175778286784,122.238070190751,43.5859783954351));
#25724=CARTESIAN_POINT('Ctrl Pts',(7.89008531462202,122.238006634921,43.584300934589));
#25725=CARTESIAN_POINT('Ctrl Pts',(7.87782318666485,122.237493013703,43.5719650959653));
#25726=CARTESIAN_POINT('Ctrl Pts',(7.8643936518537,122.237549698229,43.5584909077319));
#25727=CARTESIAN_POINT('Ctrl Pts',(7.86222207458237,122.2375,43.5563217408604));
#25728=CARTESIAN_POINT('Ctrl Pts',(7.86180395983237,122.2375,43.5559019799162));
#25729=CARTESIAN_POINT('Ctrl Pts',(7.79753717030059,122.238070190751,43.6801990080023));
#25730=CARTESIAN_POINT('Ctrl Pts',(7.795869694655,122.238006634921,43.6785165545561));
#25731=CARTESIAN_POINT('Ctrl Pts',(7.78366089805848,122.2375677537,43.6661681935589));
#25732=CARTESIAN_POINT('Ctrl Pts',(7.77028348727585,122.237504057297,43.6526067302897));
#25733=CARTESIAN_POINT('Ctrl Pts',(7.76812240830434,122.2375,43.6504214071384));
#25734=CARTESIAN_POINT('Ctrl Pts',(7.76770593974856,122.2375,43.65));
#25735=CARTESIAN_POINT('',(7.79753717030059,122.238070190751,43.6801990080023));
#25736=CARTESIAN_POINT('Ctrl Pts',(7.79753717030059,122.238070190751,43.6801990080023));
#25737=CARTESIAN_POINT('Ctrl Pts',(7.89175778286784,122.238070190751,43.5859783954351));
#25738=CARTESIAN_POINT('Ctrl Pts',(7.98597839543509,122.238070190751,43.4917577828678));
#25739=CARTESIAN_POINT('Ctrl Pts',(8.08019900800235,122.238070190751,43.3975371703006));
#25740=CARTESIAN_POINT('Ctrl Pts',(7.79753717030059,122.238070190751,43.6801990080023));
#25741=CARTESIAN_POINT('Ctrl Pts',(7.79737024716059,122.238063828476,43.6800305855052));
#25742=CARTESIAN_POINT('Ctrl Pts',(7.79720010714893,122.238057382362,43.6798589093858));
#25743=CARTESIAN_POINT('Ctrl Pts',(7.79697146331107,122.23804882687,43.6796280573389));
#25744=CARTESIAN_POINT('Ctrl Pts',(7.79671912590222,122.238039384803,43.6793732828919));
#25745=CARTESIAN_POINT('Ctrl Pts',(7.79639560212623,122.238027372131,43.6790465041629));
#25746=CARTESIAN_POINT('Ctrl Pts',(7.79597354340905,122.238012105093,43.6786200261654));
#25747=CARTESIAN_POINT('Ctrl Pts',(7.79550218532653,122.237995054761,43.6781437326003));
#25748=CARTESIAN_POINT('Ctrl Pts',(7.79490840015591,122.237973979824,43.6775435637606));
#25749=CARTESIAN_POINT('Ctrl Pts',(7.79420602224099,122.237950147598,43.6768334404111));
#25750=CARTESIAN_POINT('Ctrl Pts',(7.79331766892344,122.237920005083,43.6759352908252));
#25751=CARTESIAN_POINT('Ctrl Pts',(7.79225701215112,122.237885609635,43.6748626694998));
#25752=CARTESIAN_POINT('Ctrl Pts',(7.79111933100742,122.237851483799,43.6737118227385));
#25753=CARTESIAN_POINT('Ctrl Pts',(7.78997111967495,122.2378170421,43.6725503239297));
#25754=CARTESIAN_POINT('Ctrl Pts',(7.78874985538888,122.237783080562,43.6713146082226));
#25755=CARTESIAN_POINT('Ctrl Pts',(7.7875548864529,122.237752675088,43.6701051310899));
#25756=CARTESIAN_POINT('Ctrl Pts',(7.78666002174363,122.237729905638,43.6691994017692));
#25757=CARTESIAN_POINT('Ctrl Pts',(7.78578043150577,122.237709074602,43.6683089239629));
#25758=CARTESIAN_POINT('Ctrl Pts',(7.78493051996895,122.237690299368,43.6674482886095));
#25759=CARTESIAN_POINT('Ctrl Pts',(7.78415885587012,122.237673252684,43.6666668879864));
#25760=CARTESIAN_POINT('Ctrl Pts',(7.78341204807806,122.237657876347,43.665910483893));
#25761=CARTESIAN_POINT('Ctrl Pts',(7.7826693399016,122.237643618104,43.6651581113863));
#25762=CARTESIAN_POINT('Ctrl Pts',(7.78189239180545,122.237628702536,43.6643710534202));
#25763=CARTESIAN_POINT('Ctrl Pts',(7.78111275161813,122.237614869895,43.6635811455733));
#25764=CARTESIAN_POINT('Ctrl Pts',(7.78030566598238,122.237601821719,43.6627634000982));
#25765=CARTESIAN_POINT('Ctrl Pts',(7.77940461933911,122.237587254472,43.6618504525958));
#25766=CARTESIAN_POINT('Ctrl Pts',(7.77846992011155,122.237573726381,43.6609033701755));
#25767=CARTESIAN_POINT('Ctrl Pts',(7.77751989647083,122.237561764432,43.6599407885375));
#25768=CARTESIAN_POINT('Ctrl Pts',(7.77627787339213,122.237546125856,43.6586823476333));
#25769=CARTESIAN_POINT('Ctrl Pts',(7.77501135351555,122.237533328235,43.6573991342643));
#25770=CARTESIAN_POINT('Ctrl Pts',(7.77383386704111,122.237524073618,43.6562062234303));
#25771=CARTESIAN_POINT('Ctrl Pts',(7.77287167511409,122.237516511138,43.6552314273718));
#25772=CARTESIAN_POINT('Ctrl Pts',(7.77197216162022,122.237511277906,43.6543201973338));
#25773=CARTESIAN_POINT('Ctrl Pts',(7.77119508418019,122.237507801652,43.6535330697664));
#25774=CARTESIAN_POINT('Ctrl Pts',(7.77051841529376,122.237504774575,43.6528476493604));
#25775=CARTESIAN_POINT('Ctrl Pts',(7.76993548245554,122.237503040519,43.6522572394536));
#25776=CARTESIAN_POINT('Ctrl Pts',(7.76946159575746,122.237501974327,43.6517773349774));
#25777=CARTESIAN_POINT('Ctrl Pts',(7.76902358430123,122.237500988851,43.6513337613144));
#25778=CARTESIAN_POINT('Ctrl Pts',(7.76867922569604,122.237500559908,43.6509850931095));
#25779=CARTESIAN_POINT('Ctrl Pts',(7.76840949787714,122.237500316879,43.6507120440968));
#25780=CARTESIAN_POINT('Ctrl Pts',(7.76815889717443,122.237500091084,43.650458357715));
#25781=CARTESIAN_POINT('Ctrl Pts',(7.76797293322782,122.237500027304,43.6502701637959));
#25782=CARTESIAN_POINT('Ctrl Pts',(7.76780376677561,122.237500006124,43.6500989877796));
#25783=CARTESIAN_POINT('Ctrl Pts',(7.76777080500425,122.237500001997,43.6500656344483));
#25784=CARTESIAN_POINT('Ctrl Pts',(7.76773836991353,122.2375,43.6500328147295));
#25785=CARTESIAN_POINT('Ctrl Pts',(7.76770593974857,122.2375,43.65));
#25786=CARTESIAN_POINT('Ctrl Pts',(7.79753717030059,126.999429809249,43.6801990080023));
#25787=CARTESIAN_POINT('Ctrl Pts',(7.79586969465498,126.999493365079,43.6785165545561));
#25788=CARTESIAN_POINT('Ctrl Pts',(7.78366122669983,126.999932239882,43.6661685239879));
#25789=CARTESIAN_POINT('Ctrl Pts',(7.77028357183286,126.999995941636,43.6526068154461));
#25790=CARTESIAN_POINT('Ctrl Pts',(7.76812240830435,127.,43.6504214071384));
#25791=CARTESIAN_POINT('Ctrl Pts',(7.76770593974856,127.,43.65));
#25792=CARTESIAN_POINT('Ctrl Pts',(7.89175778286784,126.999429809249,43.5859783954351));
#25793=CARTESIAN_POINT('Ctrl Pts',(7.890085314622,126.999493365079,43.584300934589));
#25794=CARTESIAN_POINT('Ctrl Pts',(7.8778235153062,126.999932239882,43.5720062353815));
#25795=CARTESIAN_POINT('Ctrl Pts',(7.86439373641072,126.999995941636,43.5584966508682));
#25796=CARTESIAN_POINT('Ctrl Pts',(7.86222207458238,127.,43.5563217408604));
#25797=CARTESIAN_POINT('Ctrl Pts',(7.86180395983237,127.,43.5559019799162));
#25798=CARTESIAN_POINT('Ctrl Pts',(7.98597839543509,126.999429809249,43.4917577828678));
#25799=CARTESIAN_POINT('Ctrl Pts',(7.98430093458903,126.999493365079,43.490085314622));
#25800=CARTESIAN_POINT('Ctrl Pts',(7.97196542790919,127.000007018684,43.4778235153062));
#25801=CARTESIAN_POINT('Ctrl Pts',(7.9584909931402,126.999950310709,43.4643937364107));
#25802=CARTESIAN_POINT('Ctrl Pts',(7.9563217408604,127.,43.4622220745824));
#25803=CARTESIAN_POINT('Ctrl Pts',(7.95590197991619,127.,43.4618039598324));
#25804=CARTESIAN_POINT('Ctrl Pts',(8.08019900800234,126.999429809249,43.3975371703006));
#25805=CARTESIAN_POINT('Ctrl Pts',(8.07851655455605,126.999493365079,43.395869694655));
#25806=CARTESIAN_POINT('Ctrl Pts',(8.06616852398783,126.999932239882,43.3836612266998));
#25807=CARTESIAN_POINT('Ctrl Pts',(8.05260681544608,126.999995941636,43.3702835718329));
#25808=CARTESIAN_POINT('Ctrl Pts',(8.05042140713843,127.,43.3681224083043));
#25809=CARTESIAN_POINT('Ctrl Pts',(8.05,127.,43.3677059397486));
#25810=CARTESIAN_POINT('',(7.79753717030059,126.999429809249,43.6801990080023));
#25811=CARTESIAN_POINT('Ctrl Pts',(7.76770593974857,127.,43.65));
#25812=CARTESIAN_POINT('Ctrl Pts',(7.76787269880523,127.,43.650168736525));
#25813=CARTESIAN_POINT('Ctrl Pts',(7.76804267276226,126.999999960859,43.6503407294752));
#25814=CARTESIAN_POINT('Ctrl Pts',(7.76827111985223,126.999999795533,43.6505719684178));
#25815=CARTESIAN_POINT('Ctrl Pts',(7.76852323938489,126.999999613074,43.6508271691041));
#25816=CARTESIAN_POINT('Ctrl Pts',(7.76884650748516,126.99999928102,43.6511544591101));
#25817=CARTESIAN_POINT('Ctrl Pts',(7.76926826289326,126.999998436683,43.6515815512717));
#25818=CARTESIAN_POINT('Ctrl Pts',(7.76973927920159,126.999997493728,43.6520585276647));
#25819=CARTESIAN_POINT('Ctrl Pts',(7.7703326618207,126.999995895344,43.6526595049515));
#25820=CARTESIAN_POINT('Ctrl Pts',(7.77103459621293,126.999992899769,43.6533705073354));
#25821=CARTESIAN_POINT('Ctrl Pts',(7.77192235659121,126.999989111163,43.6542697363123));
#25822=CARTESIAN_POINT('Ctrl Pts',(7.77298234306036,126.999982983391,43.6553435322329));
#25823=CARTESIAN_POINT('Ctrl Pts',(7.7741193736364,126.999973630094,43.6564954718407));
#25824=CARTESIAN_POINT('Ctrl Pts',(7.77526702434735,126.999964189434,43.6576581708374));
#25825=CARTESIAN_POINT('Ctrl Pts',(7.77648776408707,126.999951463521,43.658895009794));
#25826=CARTESIAN_POINT('Ctrl Pts',(7.77768232341421,126.999936173481,43.6601053627631));
#25827=CARTESIAN_POINT('Ctrl Pts',(7.7785768692244,126.999924723534,43.6610117356427));
#25828=CARTESIAN_POINT('Ctrl Pts',(7.77945620574664,126.999911911841,43.6619027203556));
#25829=CARTESIAN_POINT('Ctrl Pts',(7.78030595164888,126.999898173663,43.6627636895377));
#25830=CARTESIAN_POINT('Ctrl Pts',(7.78107745852858,126.999885700406,43.6635453863314));
#25831=CARTESIAN_POINT('Ctrl Pts',(7.78182418239544,126.999872502733,43.6643019452788));
#25832=CARTESIAN_POINT('Ctrl Pts',(7.78256688208792,126.999858342121,43.6650543196371));
#25833=CARTESIAN_POINT('Ctrl Pts',(7.78334383167018,126.999843528486,43.6658413900361));
#25834=CARTESIAN_POINT('Ctrl Pts',(7.78412355570597,126.99982752742,43.6666311424636));
#25835=CARTESIAN_POINT('Ctrl Pts',(7.78493080552624,126.999809694323,43.6674485777698));
#25836=CARTESIAN_POINT('Ctrl Pts',(7.78583202413818,126.999789785346,43.6683611675201));
#25837=CARTESIAN_POINT('Ctrl Pts',(7.78676699423533,126.999767552882,43.6693076969476));
#25838=CARTESIAN_POINT('Ctrl Pts',(7.78771736012898,126.999743173978,43.6702695751297));
#25839=CARTESIAN_POINT('Ctrl Pts',(7.78895976345899,126.999711303693,43.6715270283533));
#25840=CARTESIAN_POINT('Ctrl Pts',(7.79022678184709,126.999675666216,43.6728089911139));
#25841=CARTESIAN_POINT('Ctrl Pts',(7.79140481190622,126.999639900927,43.6740006009271));
#25842=CARTESIAN_POINT('Ctrl Pts',(7.79236756923585,126.999610671373,43.6749744564522));
#25843=CARTESIAN_POINT('Ctrl Pts',(7.79326766127809,126.999581516184,43.6758847018358));
#25844=CARTESIAN_POINT('Ctrl Pts',(7.79404526836015,126.999555290462,43.6766709110092));
#25845=CARTESIAN_POINT('Ctrl Pts',(7.79472238065246,126.999532454046,43.6773555136934));
#25846=CARTESIAN_POINT('Ctrl Pts',(7.79530572413939,126.999511912239,43.6779451634233));
#25847=CARTESIAN_POINT('Ctrl Pts',(7.79577996677921,126.999494873465,43.6784244138505));
#25848=CARTESIAN_POINT('Ctrl Pts',(7.79621830380183,126.999479124722,43.6788673795135));
#25849=CARTESIAN_POINT('Ctrl Pts',(7.79656294241353,126.999466401456,43.6792155329299));
#25850=CARTESIAN_POINT('Ctrl Pts',(7.79683290735634,126.999456345864,43.6794881511384));
#25851=CARTESIAN_POINT('Ctrl Pts',(7.79708372688692,126.999447003396,43.6797414357699));
#25852=CARTESIAN_POINT('Ctrl Pts',(7.7972698733067,126.999439970326,43.6799293013847));
#25853=CARTESIAN_POINT('Ctrl Pts',(7.79743920767177,126.999433537031,43.6801001639553));
#25854=CARTESIAN_POINT('Ctrl Pts',(7.79747221525241,126.999432283018,43.6801334694221));
#25855=CARTESIAN_POINT('Ctrl Pts',(7.79750469524479,126.999431047036,43.6801662412452));
#25856=CARTESIAN_POINT('Ctrl Pts',(7.79753717030059,126.999429809249,43.6801990080023));
#25857=CARTESIAN_POINT('Ctrl Pts',(8.08019900800234,126.999429809249,43.3975371703006));
#25858=CARTESIAN_POINT('Ctrl Pts',(7.98597839543509,126.999429809249,43.4917577828678));
#25859=CARTESIAN_POINT('Ctrl Pts',(7.89175778286784,126.999429809249,43.5859783954351));
#25860=CARTESIAN_POINT('Ctrl Pts',(7.79753717030059,126.999429809249,43.6801990080023));
#25861=CARTESIAN_POINT('Ctrl Pts',(8.08019900800234,126.999429809249,43.3975371703006));
#25862=CARTESIAN_POINT('Ctrl Pts',(8.27787070631434,126.991962625601,43.5934491246469));
#25863=CARTESIAN_POINT('Ctrl Pts',(8.58912619963984,126.852168067061,43.9258493522423));
#25864=CARTESIAN_POINT('Ctrl Pts',(8.81677764270249,126.497776564831,44.2039080692991));
#25865=CARTESIAN_POINT('Ctrl Pts',(8.85,126.297687701072,44.25));
#25866=CARTESIAN_POINT('Ctrl Pts',(8.85,126.2,44.25));
#25867=CARTESIAN_POINT('Ctrl Pts',(7.98597839543509,126.999429809249,43.4917577828678));
#25868=CARTESIAN_POINT('Ctrl Pts',(8.1830635124252,126.991962625601,43.6882563185361));
#25869=CARTESIAN_POINT('Ctrl Pts',(8.50136725050732,126.852168067061,44.0136083013748));
#25870=CARTESIAN_POINT('Ctrl Pts',(8.74582111823467,126.497776564831,44.2748645937669));
#25871=CARTESIAN_POINT('Ctrl Pts',(8.78333333333332,126.297687701072,44.3166666666667));
#25872=CARTESIAN_POINT('Ctrl Pts',(8.78333333333332,126.2,44.3166666666667));
#25873=CARTESIAN_POINT('Ctrl Pts',(7.89175778286784,126.999429809249,43.5859783954351));
#25874=CARTESIAN_POINT('Ctrl Pts',(8.08825631853606,126.991962625601,43.7830635124252));
#25875=CARTESIAN_POINT('Ctrl Pts',(8.41360830137479,126.852168067061,44.1013672505073));
#25876=CARTESIAN_POINT('Ctrl Pts',(8.67486459376686,126.497776564831,44.3458211182347));
#25877=CARTESIAN_POINT('Ctrl Pts',(8.71666666666665,126.297687701072,44.3833333333333));
#25878=CARTESIAN_POINT('Ctrl Pts',(8.71666666666665,126.2,44.3833333333333));
#25879=CARTESIAN_POINT('Ctrl Pts',(7.79753717030059,126.999429809249,43.6801990080023));
#25880=CARTESIAN_POINT('Ctrl Pts',(7.99344912464693,126.991962625601,43.8778707063143));
#25881=CARTESIAN_POINT('Ctrl Pts',(8.32584935224227,126.852168067061,44.1891261996398));
#25882=CARTESIAN_POINT('Ctrl Pts',(8.60390806929905,126.497776564831,44.4167776427025));
#25883=CARTESIAN_POINT('Ctrl Pts',(8.64999999999998,126.297687701072,44.45));
#25884=CARTESIAN_POINT('Ctrl Pts',(8.64999999999998,126.2,44.45));
#25885=CARTESIAN_POINT('',(8.64999999999998,126.2,44.45));
#25886=CARTESIAN_POINT('Ctrl Pts',(7.79753717030059,126.999429809249,43.6801990080023));
#25887=CARTESIAN_POINT('Ctrl Pts',(7.99344912464693,126.991962625601,43.8778707063143));
#25888=CARTESIAN_POINT('Ctrl Pts',(8.32584935224227,126.852168067061,44.1891261996398));
#25889=CARTESIAN_POINT('Ctrl Pts',(8.60390806929905,126.497776564831,44.4167776427025));
#25890=CARTESIAN_POINT('Ctrl Pts',(8.64999999999998,126.297687701072,44.45));
#25891=CARTESIAN_POINT('Ctrl Pts',(8.64999999999998,126.2,44.45));
#25892=CARTESIAN_POINT('',(8.64999999999998,126.2,44.45));
#25893=CARTESIAN_POINT('Origin',(8.74999999999999,122.2375,44.35));
#25894=CARTESIAN_POINT('',(8.64999999999999,123.0375,44.45));
#25895=CARTESIAN_POINT('',(8.64999999999999,122.2375,44.45));
#25896=CARTESIAN_POINT('',(8.64999999999999,123.0375,44.45));
#25897=CARTESIAN_POINT('Ctrl Pts',(7.79753717030059,122.238070190751,43.6801990080023));
#25898=CARTESIAN_POINT('Ctrl Pts',(7.99344912464693,122.245537374399,43.8778707063143));
#25899=CARTESIAN_POINT('Ctrl Pts',(8.3258486625008,122.385332034808,44.1891258667193));
#25900=CARTESIAN_POINT('Ctrl Pts',(8.60390735497882,122.739724420659,44.4167769019277));
#25901=CARTESIAN_POINT('Ctrl Pts',(8.64999999999998,122.939812298928,44.45));
#25902=CARTESIAN_POINT('Ctrl Pts',(8.64999999999998,123.0375,44.45));
#25903=CARTESIAN_POINT('Ctrl Pts',(7.89175778286784,122.238070190751,43.5859783954351));
#25904=CARTESIAN_POINT('Ctrl Pts',(8.08825631853606,122.245537374399,43.7830635124252));
#25905=CARTESIAN_POINT('Ctrl Pts',(8.41360773057363,122.385332034808,44.1013667986465));
#25906=CARTESIAN_POINT('Ctrl Pts',(8.67486387062843,122.739724420659,44.3458203862781));
#25907=CARTESIAN_POINT('Ctrl Pts',(8.71666666666665,122.939812298928,44.3833333333333));
#25908=CARTESIAN_POINT('Ctrl Pts',(8.71666666666665,123.0375,44.3833333333333));
#25909=CARTESIAN_POINT('Ctrl Pts',(7.98597839543509,122.238070190751,43.4917577828678));
#25910=CARTESIAN_POINT('Ctrl Pts',(8.1830635124252,122.245537374399,43.6882563185361));
#25911=CARTESIAN_POINT('Ctrl Pts',(8.50136679864646,122.385332034808,44.0136077305736));
#25912=CARTESIAN_POINT('Ctrl Pts',(8.74582038627804,122.739724420659,44.2748638706285));
#25913=CARTESIAN_POINT('Ctrl Pts',(8.78333333333332,122.939812298928,44.3166666666667));
#25914=CARTESIAN_POINT('Ctrl Pts',(8.78333333333332,123.0375,44.3166666666667));
#25915=CARTESIAN_POINT('Ctrl Pts',(8.08019900800235,122.238070190751,43.3975371703006));
#25916=CARTESIAN_POINT('Ctrl Pts',(8.27787070631434,122.245537374399,43.5934491246469));
#25917=CARTESIAN_POINT('Ctrl Pts',(8.5891258667193,122.385332034808,43.9258486625008));
#25918=CARTESIAN_POINT('Ctrl Pts',(8.81677690192765,122.739724420659,44.2039073549789));
#25919=CARTESIAN_POINT('Ctrl Pts',(8.85,122.939812298928,44.25));
#25920=CARTESIAN_POINT('Ctrl Pts',(8.85,123.0375,44.25));
#25921=CARTESIAN_POINT('Ctrl Pts',(8.64999999999998,123.0375,44.45));
#25922=CARTESIAN_POINT('Ctrl Pts',(8.64999999999998,122.939812298928,44.45));
#25923=CARTESIAN_POINT('Ctrl Pts',(8.60390735497882,122.739724420659,44.4167769019277));
#25924=CARTESIAN_POINT('Ctrl Pts',(8.3258486625008,122.385332034808,44.1891258667193));
#25925=CARTESIAN_POINT('Ctrl Pts',(7.99344912464693,122.245537374399,43.8778707063143));
#25926=CARTESIAN_POINT('Ctrl Pts',(7.79753717030059,122.238070190751,43.6801990080023));
#25927=CARTESIAN_POINT('Origin',(-48.3,123.0375,43.65));
#25928=CARTESIAN_POINT('',(-48.3,123.0375,44.45));
#25929=CARTESIAN_POINT('Origin',(-67.35,122.2375,44.45));
#25930=CARTESIAN_POINT('',(-48.3,126.2,44.45));
#25931=CARTESIAN_POINT('Origin',(-48.3,126.2,43.65));
#25932=CARTESIAN_POINT('Origin',(-10.2,126.2,-107.15));
#25933=CARTESIAN_POINT('',(-10.2,126.2,-107.95));
#25934=CARTESIAN_POINT('Origin',(8.85,122.2375,-107.95));
#25935=CARTESIAN_POINT('',(-10.2,123.0375,-107.95));
#25936=CARTESIAN_POINT('Origin',(-10.2,123.0375,-107.15));
#32285=UNCERTAINTY_MEASURE_WITH_UNIT(LENGTH_MEASURE(0.01),#32310,
'DISTANCE_ACCURACY_VALUE',
'Maximum model space distance between geometric entities at asserted c
onnectivities');
#32293=UNCERTAINTY_MEASURE_WITH_UNIT(LENGTH_MEASURE(0.01),#32310,
'DISTANCE_ACCURACY_VALUE',
'Maximum model space distance between geometric entities at asserted c
onnectivities');
#32301=(
GEOMETRIC_REPRESENTATION_CONTEXT(3)
GLOBAL_UNCERTAINTY_ASSIGNED_CONTEXT((#32285))
GLOBAL_UNIT_ASSIGNED_CONTEXT((#32310,#32312,#32313))
REPRESENTATION_CONTEXT('','3D')
);
#32309=(
GEOMETRIC_REPRESENTATION_CONTEXT(3)
GLOBAL_UNCERTAINTY_ASSIGNED_CONTEXT((#32293))
GLOBAL_UNIT_ASSIGNED_CONTEXT((#32310,#32312,#32313))
REPRESENTATION_CONTEXT('','3D')
);
#32310=(
LENGTH_UNIT()
NAMED_UNIT(*)
SI_UNIT(.MILLI.,.METRE.)
);
#32312=(
NAMED_UNIT(*)
PLANE_ANGLE_UNIT()
SI_UNIT($,.RADIAN.)
);
#32313=(
NAMED_UNIT(*)
SI_UNIT($,.STERADIAN.)
SOLID_ANGLE_UNIT()
);
#32321=SHAPE_DEFINITION_REPRESENTATION(#32336,#32368);
#32336=PRODUCT_DEFINITION_SHAPE('',$,#32384);
#32368=SHAPE_REPRESENTATION('',(#14413),#32301);
#32376=PRODUCT_DEFINITION_CONTEXT('part definition',#32423,'design');
#32384=PRODUCT_DEFINITION('2026-10-25-00-35-17-868',
'07_Inner_Door_Plate_3in',#32399,#32376);
#32399=PRODUCT_DEFINITION_FORMATION('',$,#32432);
#32423=APPLICATION_CONTEXT(
'Core Data for Automotive Mechanical Design Process');
#32424=PRODUCT_CONTEXT('part definition',#32423,'mechanical');
#32432=PRODUCT('2026-10-25-00-35-17-868','07_Inner_Door_Plate_3in',$,(#32424));
#32489=COLOUR_RGB('Sky Blue',0.24,0.69,0.87);
#32490=FILL_AREA_STYLE_COLOUR('',#32489);
#32491=FILL_AREA_STYLE('',(#32490));
#32492=SURFACE_STYLE_FILL_AREA(#32491);
#32493=SURFACE_SIDE_STYLE('',(#32492));
#32494=SURFACE_STYLE_USAGE(.BOTH.,#32493);
#32495=PRESENTATION_STYLE_ASSIGNMENT((#32494));
ENDSEC;
END-ISO-10303-21;
